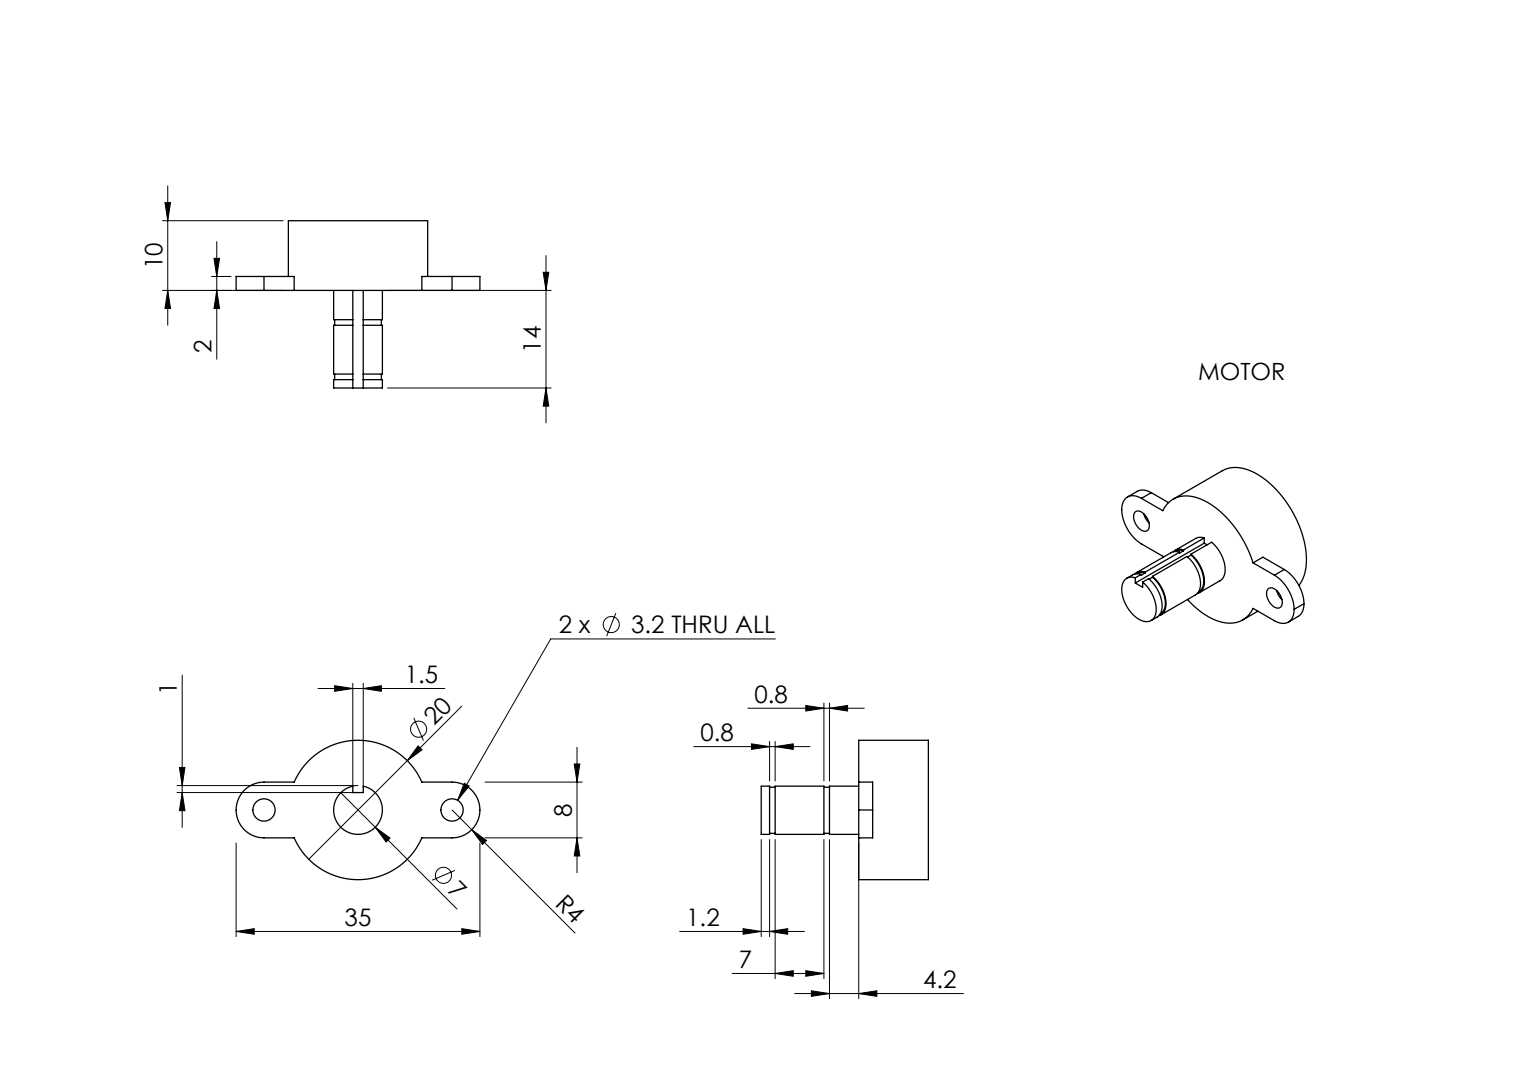
ISO-10303-21;
HEADER;
FILE_DESCRIPTION (('STEP AP214'),
    '1' );
FILE_NAME ('motor.step',
    '2026-10-26T05:17:54',
    ( '' ),
    ( '' ),
    'SwSTEP 2.0',
    'SolidWorks 2026',
    '' );
FILE_SCHEMA (( 'AUTOMOTIVE_DESIGN' ));
ENDSEC;

DATA;
#3=ORIENTED_EDGE ( 'NONE', *, *, #1888, .T. ) ;
#13=CARTESIAN_POINT ( 'NONE',  ( 19.89999999999999503, 90.00000000000000000, -8.000000000000000000 ) ) ;
#19=EDGE_CURVE ( 'NONE', #6404, #5937, #10592, .T. ) ;
#21=CIRCLE ( 'NONE', #6519, 3.500000000000003109 ) ;
#29=VERTEX_POINT ( 'NONE', #4640 ) ;
#47=ORIENTED_EDGE ( 'NONE', *, *, #5628, .T. ) ;
#48=EDGE_CURVE ( 'NONE', #8414, #6329, #6123, .T. ) ;
#56=PLANE ( 'NONE',  #9383 ) ;
#67=DIRECTION ( 'NONE',  ( 0.000000000000000000, 1.000000000000000000, 0.000000000000000000 ) ) ;
#70=LINE ( 'NONE', #8139, #12259 ) ;
#71=ORIENTED_EDGE ( 'NONE', *, *, #3443, .T. ) ;
#83=AXIS2_PLACEMENT_3D ( 'NONE', #3379, #1527, #7355 ) ;
#88=ORIENTED_EDGE ( 'NONE', *, *, #8982, .F. ) ;
#103=CIRCLE ( 'NONE', #2000, 3.500000000000003109 ) ;
#107=DIRECTION ( 'NONE',  ( -1.000000000000000000, 0.000000000000000000, 0.000000000000000000 ) ) ;
#115=VECTOR ( 'NONE', #5469, 1000.000000000000000 ) ;
#121=DIRECTION ( 'NONE',  ( -0.8665440819333538602, -0.4991005450470686888, -4.805464830191153728E-17 ) ) ;
#126=ORIENTED_EDGE ( 'NONE', *, *, #19, .T. ) ;
#142=DIRECTION ( 'NONE',  ( -0.000000000000000000, 0.000000000000000000, -1.000000000000000000 ) ) ;
#145=CARTESIAN_POINT ( 'NONE',  ( 34.25000000000000000, 92.49999999999998579, 4.800000000000000711 ) ) ;
#151=ORIENTED_EDGE ( 'NONE', *, *, #731, .F. ) ;
#165=AXIS2_PLACEMENT_3D ( 'NONE', #5058, #1689, #12557 ) ;
#166=LINE ( 'NONE', #6266, #6322 ) ;
#170=PRODUCT_DEFINITION_CONTEXT ( 'detailed design', #1838, 'design' ) ;
#181=ORIENTED_EDGE ( 'NONE', *, *, #7547, .F. ) ;
#185=DIRECTION ( 'NONE',  ( -0.3553942263724512163, 0.9347165045408831752, 0.000000000000000000 ) ) ;
#187=DIRECTION ( 'NONE',  ( -0.000000000000000000, -0.000000000000000000, -1.000000000000000000 ) ) ;
#191=VERTEX_POINT ( 'NONE', #1882 ) ;
#216=VERTEX_POINT ( 'NONE', #11026 ) ;
#237=VERTEX_POINT ( 'NONE', #12343 ) ;
#250=CARTESIAN_POINT ( 'NONE',  ( 50.09999999999995168, 90.00000000000000000, -10.00000000000000000 ) ) ;
#251=FACE_OUTER_BOUND ( 'NONE', #2972, .T. ) ;
#252=VERTEX_POINT ( 'NONE', #288 ) ;
#285=DIRECTION ( 'NONE',  ( 0.000000000000000000, 0.000000000000000000, -1.000000000000000000 ) ) ;
#288=CARTESIAN_POINT ( 'NONE',  ( 50.09999999999995168, 90.00000000000000000, -8.000000000000000000 ) ) ;
#292=CARTESIAN_POINT ( 'NONE',  ( 35.00000000000000000, 90.00000000000000000, 4.000000000000000000 ) ) ;
#294=VERTEX_POINT ( 'NONE', #6118 ) ;
#297=CARTESIAN_POINT ( 'NONE',  ( 52.49999999999996447, 94.00000000000000000, -10.00000000000000000 ) ) ;
#299=ORIENTED_EDGE ( 'NONE', *, *, #12486, .F. ) ;
#310=EDGE_CURVE ( 'NONE', #8511, #12562, #11290, .T. ) ;
#337=DIRECTION ( 'NONE',  ( -0.000000000000000000, -0.000000000000000000, -1.000000000000000000 ) ) ;
#341=DIRECTION ( 'NONE',  ( -0.3262398754384822630, 0.9452870165584014162, 0.000000000000000000 ) ) ;
#358=AXIS2_PLACEMENT_3D ( 'NONE', #3613, #12439, #9423 ) ;
#370=VERTEX_POINT ( 'NONE', #1148 ) ;
#387=ORIENTED_EDGE ( 'NONE', *, *, #9281, .T. ) ;
#393=CIRCLE ( 'NONE', #7723, 4.000000000000003553 ) ;
#400=AXIS2_PLACEMENT_3D ( 'NONE', #292, #2539, #8422 ) ;
#401=CARTESIAN_POINT ( 'NONE',  ( 48.49999999999995737, 94.00000000000000000, -8.000000000000000000 ) ) ;
#403=CARTESIAN_POINT ( 'NONE',  ( 35.00000000000000000, 90.00000000000000000, 4.800000000000000711 ) ) ;
#407=ADVANCED_FACE ( 'NONE', ( #2595 ), #7436, .F. ) ;
#408=VERTEX_POINT ( 'NONE', #12543 ) ;
#409=CARTESIAN_POINT ( 'NONE',  ( 25.00000000000000000, 90.00000000000000000, -10.00000000000000000 ) ) ;
#412=ORIENTED_EDGE ( 'NONE', *, *, #1216, .T. ) ;
#430=DIRECTION ( 'NONE',  ( -5.624500927088228034E-17, 1.370729058197317775E-18, 1.000000000000000000 ) ) ;
#431=AXIS2_PLACEMENT_3D ( 'NONE', #2573, #8714, #3560 ) ;
#447=DIRECTION ( 'NONE',  ( 0.000000000000000000, 0.000000000000000000, -1.000000000000000000 ) ) ;
#457=AXIS2_PLACEMENT_3D ( 'NONE', #11629, #9541, #8624 ) ;
#463=DIRECTION ( 'NONE',  ( -0.000000000000000000, -0.000000000000000000, 1.000000000000000000 ) ) ;
#485=VERTEX_POINT ( 'NONE', #3968 ) ;
#499=AXIS2_PLACEMENT_3D ( 'NONE', #6594, #5619, #11504 ) ;
#507=LINE ( 'NONE', #4515, #8154 ) ;
#531=EDGE_CURVE ( 'NONE', #3957, #12821, #1005, .T. ) ;
#535=DIRECTION ( 'NONE',  ( -5.624500927088228034E-17, 1.370729058197317968E-18, 1.000000000000000000 ) ) ;
#537=LINE ( 'NONE', #1464, #10952 ) ;
#543=ORIENTED_EDGE ( 'NONE', *, *, #11638, .F. ) ;
#557=ORIENTED_EDGE ( 'NONE', *, *, #7447, .F. ) ;
#565=FACE_OUTER_BOUND ( 'NONE', #1775, .T. ) ;
#575=ORIENTED_EDGE ( 'NONE', *, *, #4120, .F. ) ;
#578=ORIENTED_EDGE ( 'NONE', *, *, #7988, .T. ) ;
#581=AXIS2_PLACEMENT_3D ( 'NONE', #6283, #2043, #10989 ) ;
#583=DIRECTION ( 'NONE',  ( -1.000000000000000000, 0.000000000000000000, 0.000000000000000000 ) ) ;
#600=AXIS2_PLACEMENT_3D ( 'NONE', #4155, #337, #1325 ) ;
#624=AXIS2_PLACEMENT_3D ( 'NONE', #12004, #1206, #5133 ) ;
#636=CARTESIAN_POINT ( 'NONE',  ( 35.75000000000000711, 92.49999999999998579, -3.000000000000000000 ) ) ;
#644=ORIENTED_EDGE ( 'NONE', *, *, #5801, .F. ) ;
#650=ORIENTED_EDGE ( 'NONE', *, *, #2075, .F. ) ;
#655=VERTEX_POINT ( 'NONE', #9185 ) ;
#660=FACE_OUTER_BOUND ( 'NONE', #1254, .T. ) ;
#668=DIRECTION ( 'NONE',  ( 0.000000000000000000, 1.000000000000000000, -1.370729058197317775E-18 ) ) ;
#675=DIRECTION ( 'NONE',  ( 5.624500927088228034E-17, -1.370729058197317775E-18, -1.000000000000000000 ) ) ;
#681=VERTEX_POINT ( 'NONE', #7030 ) ;
#693=EDGE_CURVE ( 'NONE', #12083, #4963, #12636, .T. ) ;
#699=CLOSED_SHELL ( 'NONE', ( #4681, #2294, #5712, #12137, #6395, #6284, #10454, #6271, #7033, #8769, #9664, #6996, #3078, #6506, #5758, #9872, #10478, #5588, #2469, #1397, #4829, #5175, #6473, #11028, #2843, #8926, #11939, #3918, #407, #9755, #9220, #11801, #9117, #7996, #2544, #5940, #1715, #12395, #866, #5366, #1669, #7054, #12542, #2318, #6182, #10197, #10507 ) ) ;
#705=EDGE_CURVE ( 'NONE', #12083, #370, #10296, .T. ) ;
#706=ORIENTED_EDGE ( 'NONE', *, *, #3432, .T. ) ;
#719=FACE_OUTER_BOUND ( 'NONE', #6790, .T. ) ;
#721=CIRCLE ( 'NONE', #499, 10.00000000000000178 ) ;
#731=EDGE_CURVE ( 'NONE', #10645, #11257, #10099, .T. ) ;
#738=CARTESIAN_POINT ( 'NONE',  ( 31.50000000000000000, 90.00000000000000000, -8.000000000000000000 ) ) ;
#769=CARTESIAN_POINT ( 'NONE',  ( 34.25000000000000000, 92.49999999999998579, 4.000000000000000000 ) ) ;
#777=DIRECTION ( 'NONE',  ( 0.4719909656437444867, -0.8816033849473842166, 0.000000000000000000 ) ) ;
#781=ORIENTED_EDGE ( 'NONE', *, *, #10591, .T. ) ;
#785=CIRCLE ( 'NONE', #2474, 3.500000000000003109 ) ;
#796=DIRECTION ( 'NONE',  ( -0.3262398754384820410, 0.9452870165584015272, 0.000000000000000000 ) ) ;
#806=ORIENTED_EDGE ( 'NONE', *, *, #5628, .F. ) ;
#811=LINE ( 'NONE', #3838, #1160 ) ;
#823=DIRECTION ( 'NONE',  ( -0.000000000000000000, 0.000000000000000000, 1.000000000000000000 ) ) ;
#839=AXIS2_PLACEMENT_3D ( 'NONE', #8214, #8409, #1467 ) ;
#840=CARTESIAN_POINT ( 'NONE',  ( 19.89999999999999503, 90.00000000000000000, -10.00000000000000000 ) ) ;
#841=EDGE_CURVE ( 'NONE', #3363, #7515, #10366, .T. ) ;
#843=LINE ( 'NONE', #2699, #6376 ) ;
#849=ORIENTED_EDGE ( 'NONE', *, *, #1595, .F. ) ;
#866=ADVANCED_FACE ( 'NONE', ( #2390 ), #7550, .T. ) ;
#867=EDGE_CURVE ( 'NONE', #12412, #10917, #6497, .T. ) ;
#869=LINE ( 'NONE', #9776, #11647 ) ;
#879=AXIS2_PLACEMENT_3D ( 'NONE', #12949, #12888, #6862 ) ;
#885=CARTESIAN_POINT ( 'NONE',  ( 21.49999999999998579, 90.00000000000000000, -10.00000000000000000 ) ) ;
#888=ORIENTED_EDGE ( 'NONE', *, *, #8720, .T. ) ;
#898=( GEOMETRIC_REPRESENTATION_CONTEXT ( 3 ) GLOBAL_UNCERTAINTY_ASSIGNED_CONTEXT ( ( #6165 ) ) GLOBAL_UNIT_ASSIGNED_CONTEXT ( ( #7994, #6701, #11056 ) ) REPRESENTATION_CONTEXT ( 'NONE', 'WORKASPACE' ) );
#914=VECTOR ( 'NONE', #1674, 1000.000000000000000 ) ;
#917=EDGE_CURVE ( 'NONE', #12608, #8631, #537, .T. ) ;
#931=EDGE_CURVE ( 'NONE', #1668, #8414, #9445, .T. ) ;
#934=AXIS2_PLACEMENT_3D ( 'NONE', #10445, #11553, #3520 ) ;
#938=EDGE_CURVE ( 'NONE', #252, #6072, #5110, .T. ) ;
#971=DIRECTION ( 'NONE',  ( -0.000000000000000000, -0.000000000000000000, -1.000000000000000000 ) ) ;
#980=CIRCLE ( 'NONE', #9970, 4.000000000000000000 ) ;
#981=DIRECTION ( 'NONE',  ( -0.000000000000000000, -0.000000000000000000, 1.000000000000000000 ) ) ;
#993=DIRECTION ( 'NONE',  ( 1.000000000000000000, 0.000000000000000000, 0.000000000000000000 ) ) ;
#1005=LINE ( 'NONE', #10886, #10745 ) ;
#1012=AXIS2_PLACEMENT_3D ( 'NONE', #9319, #2389, #5259 ) ;
#1020=DIRECTION ( 'NONE',  ( 0.000000000000000000, 0.000000000000000000, 1.000000000000000000 ) ) ;
#1026=ORIENTED_EDGE ( 'NONE', *, *, #5667, .T. ) ;
#1042=VECTOR ( 'NONE', #2332, 1000.000000000000000 ) ;
#1043=CARTESIAN_POINT ( 'NONE',  ( 17.49999999999998579, 90.00000000000002842, -8.000000000000000000 ) ) ;
#1072=DIRECTION ( 'NONE',  ( -1.000000000000000000, 0.000000000000000000, 0.000000000000000000 ) ) ;
#1074=ORIENTED_EDGE ( 'NONE', *, *, #9115, .T. ) ;
#1087=CIRCLE ( 'NONE', #457, 1.599999999999990319 ) ;
#1099=ORIENTED_EDGE ( 'NONE', *, *, #12396, .F. ) ;
#1124=DIRECTION ( 'NONE',  ( 0.000000000000000000, 1.000000000000000000, -1.370729058197317775E-18 ) ) ;
#1126=ORIENTED_EDGE ( 'NONE', *, *, #8124, .T. ) ;
#1128=FACE_OUTER_BOUND ( 'NONE', #1276, .T. ) ;
#1136=LINE ( 'NONE', #145, #7950 ) ;
#1141=AXIS2_PLACEMENT_3D ( 'NONE', #1428, #3600, #12425 ) ;
#1148=CARTESIAN_POINT ( 'NONE',  ( 33.90709641728108892, 93.16671150547063007, 4.000000000000000000 ) ) ;
#1158=EDGE_LOOP ( 'NONE', ( #7100, #8756, #5861, #11911, #2951, #5490, #7151, #3080, #5486, #5090, #126, #8702 ) ) ;
#1160=VECTOR ( 'NONE', #10888, 1000.000000000000000 ) ;
#1166=EDGE_LOOP ( 'NONE', ( #412, #7388 ) ) ;
#1169=PRODUCT_CONTEXT ( 'NONE', #10180, 'mechanical' ) ;
#1180=LINE ( 'NONE', #250, #9978 ) ;
#1183=CARTESIAN_POINT ( 'NONE',  ( 35.00000000000000000, 90.00000000000000000, 6.000000000000000000 ) ) ;
#1206=DIRECTION ( 'NONE',  ( -0.000000000000000000, -0.000000000000000000, -1.000000000000000000 ) ) ;
#1211=CARTESIAN_POINT ( 'NONE',  ( 34.25000000000000000, 93.41869858279433458, 4.800000000000000711 ) ) ;
#1216=EDGE_CURVE ( 'NONE', #1668, #4783, #721, .T. ) ;
#1220=CARTESIAN_POINT ( 'NONE',  ( 35.00000000000000000, 90.00000000000000000, 4.000000000000000000 ) ) ;
#1222=ORIENTED_EDGE ( 'NONE', *, *, #48, .F. ) ;
#1223=DIRECTION ( 'NONE',  ( 5.624500927088228034E-17, -1.370729058197317775E-18, -1.000000000000000000 ) ) ;
#1231=ORIENTED_EDGE ( 'NONE', *, *, #5801, .T. ) ;
#1235=CIRCLE ( 'NONE', #10439, 3.349999999999995204 ) ;
#1236=DIRECTION ( 'NONE',  ( 0.000000000000000000, 0.000000000000000000, 1.000000000000000000 ) ) ;
#1254=EDGE_LOOP ( 'NONE', ( #7238, #10734, #387, #7725 ) ) ;
#1257=AXIS2_PLACEMENT_3D ( 'NONE', #12940, #5020, #6193 ) ;
#1274=DIRECTION ( 'NONE',  ( -0.9549484348006339607, -0.2967717757331703732, 0.000000000000000000 ) ) ;
#1276=EDGE_LOOP ( 'NONE', ( #4208, #71, #3279, #2759 ) ) ;
#1289=LINE ( 'NONE', #6262, #7232 ) ;
#1296=ORIENTED_EDGE ( 'NONE', *, *, #3497, .F. ) ;
#1299=CARTESIAN_POINT ( 'NONE',  ( 52.49999999999996447, 90.00000000000000000, -10.00000000000000000 ) ) ;
#1311=DIRECTION ( 'NONE',  ( 5.624500927088228034E-17, -1.370729058197317775E-18, -1.000000000000000000 ) ) ;
#1325=DIRECTION ( 'NONE',  ( -1.000000000000000000, 0.000000000000000000, 0.000000000000000000 ) ) ;
#1335=ORIENTED_EDGE ( 'NONE', *, *, #5063, .F. ) ;
#1343=LINE ( 'NONE', #9197, #12715 ) ;
#1348=FACE_OUTER_BOUND ( 'NONE', #2904, .T. ) ;
#1353=VERTEX_POINT ( 'NONE', #7583 ) ;
#1357=CIRCLE ( 'NONE', #12227, 3.500000000000003109 ) ;
#1363=ORIENTED_EDGE ( 'NONE', *, *, #917, .F. ) ;
#1371=DIRECTION ( 'NONE',  ( 0.000000000000000000, -0.000000000000000000, 1.000000000000000000 ) ) ;
#1372=ORIENTED_EDGE ( 'NONE', *, *, #6536, .T. ) ;
#1381=ORIENTED_EDGE ( 'NONE', *, *, #6577, .T. ) ;
#1392=DIRECTION ( 'NONE',  ( -0.000000000000000000, -0.000000000000000000, -1.000000000000000000 ) ) ;
#1397=ADVANCED_FACE ( 'NONE', ( #2997 ), #11830, .F. ) ;
#1405=DIRECTION ( 'NONE',  ( -1.000000000000000000, 0.000000000000000000, 0.000000000000000000 ) ) ;
#1414=DIRECTION ( 'NONE',  ( -1.000000000000000000, 0.000000000000000000, 0.000000000000000000 ) ) ;
#1428=CARTESIAN_POINT ( 'NONE',  ( 35.00000000000000000, 90.00000000000000000, 4.800000000000000711 ) ) ;
#1443=AXIS2_PLACEMENT_3D ( 'NONE', #5383, #142, #7228 ) ;
#1448=ORIENTED_EDGE ( 'NONE', *, *, #3532, .F. ) ;
#1464=CARTESIAN_POINT ( 'NONE',  ( 34.25000000000000000, 92.49999999999998579, -3.799999999999999378 ) ) ;
#1467=DIRECTION ( 'NONE',  ( 1.000000000000000000, 0.000000000000000000, 0.000000000000000000 ) ) ;
#1469=ORIENTED_EDGE ( 'NONE', *, *, #11376, .T. ) ;
#1487=DIRECTION ( 'NONE',  ( -0.3262398754384822630, 0.9452870165584014162, 0.000000000000000000 ) ) ;
#1489=EDGE_CURVE ( 'NONE', #191, #4989, #6156, .T. ) ;
#1503=EDGE_CURVE ( 'NONE', #6072, #252, #4507, .T. ) ;
#1527=DIRECTION ( 'NONE',  ( 0.000000000000000000, 0.000000000000000000, -1.000000000000000000 ) ) ;
#1530=CARTESIAN_POINT ( 'NONE',  ( 25.83484861008832567, 94.00000000000000000, -18.00000000000000355 ) ) ;
#1552=DIRECTION ( 'NONE',  ( 0.000000000000000000, -0.000000000000000000, 1.000000000000000000 ) ) ;
#1554=DIRECTION ( 'NONE',  ( -0.000000000000000000, -0.000000000000000000, 1.000000000000000000 ) ) ;
#1567=ORIENTED_EDGE ( 'NONE', *, *, #1605, .F. ) ;
#1570=LINE ( 'NONE', #2625, #7138 ) ;
#1572=ORIENTED_EDGE ( 'NONE', *, *, #5667, .F. ) ;
#1577=ORIENTED_EDGE ( 'NONE', *, *, #9238, .F. ) ;
#1595=EDGE_CURVE ( 'NONE', #191, #7314, #8165, .T. ) ;
#1605=EDGE_CURVE ( 'NONE', #2737, #4447, #9508, .T. ) ;
#1612=CARTESIAN_POINT ( 'NONE',  ( 34.25000000000000000, 92.49999999999998579, -9.802775637731997449 ) ) ;
#1624=CARTESIAN_POINT ( 'NONE',  ( 32.09707732552327286, 88.32801317409231956, -3.800000000000000266 ) ) ;
#1625=EDGE_CURVE ( 'NONE', #8631, #6452, #1357, .T. ) ;
#1630=ORIENTED_EDGE ( 'NONE', *, *, #1964, .F. ) ;
#1637=EDGE_CURVE ( 'NONE', #12207, #7597, #3676, .T. ) ;
#1641=DIRECTION ( 'NONE',  ( -0.000000000000000000, -0.000000000000000000, -1.000000000000000000 ) ) ;
#1656=VECTOR ( 'NONE', #1725, 1000.000000000000000 ) ;
#1658=AXIS2_PLACEMENT_3D ( 'NONE', #12179, #4204, #2310 ) ;
#1661=LINE ( 'NONE', #6561, #5018 ) ;
#1668=VERTEX_POINT ( 'NONE', #7174 ) ;
#1669=ADVANCED_FACE ( 'NONE', ( #1348 ), #2217, .F. ) ;
#1674=DIRECTION ( 'NONE',  ( 0.000000000000000000, -1.000000000000000000, 1.370729058197317775E-18 ) ) ;
#1689=DIRECTION ( 'NONE',  ( -5.624500927088228034E-17, 1.370729058197317968E-18, 1.000000000000000000 ) ) ;
#1694=VERTEX_POINT ( 'NONE', #4753 ) ;
#1706=DIRECTION ( 'NONE',  ( 0.000000000000000000, 0.000000000000000000, -1.000000000000000000 ) ) ;
#1712=CARTESIAN_POINT ( 'NONE',  ( 34.25000000000000000, 93.41869858279433458, 4.000000000000000000 ) ) ;
#1715=ADVANCED_FACE ( 'NONE', ( #5601 ), #9718, .F. ) ;
#1724=EDGE_CURVE ( 'NONE', #6762, #12412, #3252, .T. ) ;
#1725=DIRECTION ( 'NONE',  ( -0.000000000000000000, -0.000000000000000000, -1.000000000000000000 ) ) ;
#1735=VERTEX_POINT ( 'NONE', #3711 ) ;
#1746=EDGE_LOOP ( 'NONE', ( #9745, #2949, #5116, #2908, #10024, #12272 ) ) ;
#1754=ORIENTED_EDGE ( 'NONE', *, *, #5511, .F. ) ;
#1767=CARTESIAN_POINT ( 'NONE',  ( 35.00000000000000000, 90.00000000000000000, -3.000000000000000000 ) ) ;
#1769=AXIS2_PLACEMENT_3D ( 'NONE', #403, #2652, #8472 ) ;
#1774=DIRECTION ( 'NONE',  ( -0.3262398754384820410, 0.9452870165584015272, 0.000000000000000000 ) ) ;
#1775=EDGE_LOOP ( 'NONE', ( #3619, #4581, #9169, #3707 ) ) ;
#1777=DIRECTION ( 'NONE',  ( -0.000000000000000000, -0.000000000000000000, -1.000000000000000000 ) ) ;
#1789=VECTOR ( 'NONE', #4577, 1000.000000000000000 ) ;
#1797=ORIENTED_EDGE ( 'NONE', *, *, #731, .T. ) ;
#1816=DIRECTION ( 'NONE',  ( -5.624500927088228034E-17, 1.370729058197317775E-18, 1.000000000000000000 ) ) ;
#1817=CARTESIAN_POINT ( 'NONE',  ( 35.00000000000000000, 90.00000000000000000, 4.000000000000000000 ) ) ;
#1828=ORIENTED_EDGE ( 'NONE', *, *, #4046, .T. ) ;
#1830=VERTEX_POINT ( 'NONE', #5004 ) ;
#1838=APPLICATION_CONTEXT ( 'automotive_design' ) ;
#1870=CIRCLE ( 'NONE', #9177, 3.350000000000003642 ) ;
#1875=EDGE_CURVE ( 'NONE', #10645, #1694, #6587, .T. ) ;
#1877=VECTOR ( 'NONE', #11062, 1000.000000000000000 ) ;
#1882=CARTESIAN_POINT ( 'NONE',  ( 38.50000000000000711, 90.00000000000000000, 4.000000000000000000 ) ) ;
#1883=CIRCLE ( 'NONE', #2727, 4.000000000000000000 ) ;
#1888=EDGE_CURVE ( 'NONE', #408, #2123, #103, .T. ) ;
#1914=ORIENTED_EDGE ( 'NONE', *, *, #8639, .T. ) ;
#1920=FACE_OUTER_BOUND ( 'NONE', #12041, .T. ) ;
#1936=ORIENTED_EDGE ( 'NONE', *, *, #8160, .F. ) ;
#1950=ORIENTED_EDGE ( 'NONE', *, *, #9238, .T. ) ;
#1955=ORIENTED_EDGE ( 'NONE', *, *, #1605, .T. ) ;
#1956=CARTESIAN_POINT ( 'NONE',  ( 34.25000000000000000, 93.41869858279433458, -3.000000000000000888 ) ) ;
#1959=STYLED_ITEM ( 'NONE', ( #8256 ), #8095 ) ;
#1964=EDGE_CURVE ( 'NONE', #2737, #10645, #811, .T. ) ;
#1968=DIRECTION ( 'NONE',  ( 0.000000000000000000, 0.000000000000000000, -1.000000000000000000 ) ) ;
#1981=ORIENTED_EDGE ( 'NONE', *, *, #4046, .F. ) ;
#1984=CARTESIAN_POINT ( 'NONE',  ( 34.25000000000000000, 93.26496554346289258, 4.800000000000000711 ) ) ;
#1988=DIRECTION ( 'NONE',  ( -5.624500927088228034E-17, 1.370729058197317775E-18, 1.000000000000000000 ) ) ;
#2000=AXIS2_PLACEMENT_3D ( 'NONE', #9846, #3907, #7032 ) ;
#2005=CARTESIAN_POINT ( 'NONE',  ( 31.50000000000000000, 90.00000000000000000, 6.000000000000000000 ) ) ;
#2010=DIRECTION ( 'NONE',  ( -0.000000000000000000, -0.000000000000000000, -1.000000000000000000 ) ) ;
#2023=DIRECTION ( 'NONE',  ( -0.3262398754384822630, 0.9452870165584014162, 0.000000000000000000 ) ) ;
#2026=DIRECTION ( 'NONE',  ( 5.624500927088228034E-17, -1.370729058197317775E-18, -1.000000000000000000 ) ) ;
#2037=EDGE_LOOP ( 'NONE', ( #575, #9948, #11098, #3, #1099, #1754 ) ) ;
#2043=DIRECTION ( 'NONE',  ( 0.000000000000000000, 0.000000000000000000, -1.000000000000000000 ) ) ;
#2055=LINE ( 'NONE', #7149, #8796 ) ;
#2064=DIRECTION ( 'NONE',  ( 0.000000000000000000, -0.000000000000000000, 1.000000000000000000 ) ) ;
#2068=DIRECTION ( 'NONE',  ( -1.000000000000000000, 0.000000000000000000, -0.000000000000000000 ) ) ;
#2074=CIRCLE ( 'NONE', #1443, 4.000000000000000000 ) ;
#2075=EDGE_CURVE ( 'NONE', #3524, #1694, #2330, .T. ) ;
#2091=DIRECTION ( 'NONE',  ( 0.4719909656437444867, -0.8816033849473842166, 0.000000000000000000 ) ) ;
#2103=ORIENTED_EDGE ( 'NONE', *, *, #10688, .T. ) ;
#2108=CARTESIAN_POINT ( 'NONE',  ( 35.00000000000000000, 90.00000000000000000, 4.800000000000000711 ) ) ;
#2110=DIRECTION ( 'NONE',  ( -0.8665440819333538602, -0.4991005450470686888, -4.805464830191153728E-17 ) ) ;
#2123=VERTEX_POINT ( 'NONE', #4227 ) ;
#2131=AXIS2_PLACEMENT_3D ( 'NONE', #7843, #10790, #2023 ) ;
#2133=FACE_OUTER_BOUND ( 'NONE', #10319, .T. ) ;
#2137=ORIENTED_EDGE ( 'NONE', *, *, #5023, .F. ) ;
#2145=CARTESIAN_POINT ( 'NONE',  ( 35.00000000000000000, 90.00000000000000000, -3.799999999999999378 ) ) ;
#2147=ORIENTED_EDGE ( 'NONE', *, *, #12555, .F. ) ;
#2148=AXIS2_PLACEMENT_3D ( 'NONE', #11822, #5987, #2990 ) ;
#2152=EDGE_LOOP ( 'NONE', ( #6828, #7770, #5880, #2183, #806, #9980 ) ) ;
#2176=CARTESIAN_POINT ( 'NONE',  ( 21.49999999999998579, 86.00000000000000000, -10.00000000000000000 ) ) ;
#2177=VERTEX_POINT ( 'NONE', #3572 ) ;
#2183=ORIENTED_EDGE ( 'NONE', *, *, #9832, .F. ) ;
#2185=DIRECTION ( 'NONE',  ( 0.4719909656437442647, -0.8816033849473842166, 2.775557561595757269E-17 ) ) ;
#2207=CARTESIAN_POINT ( 'NONE',  ( 48.49999999999995737, 90.00000000000000000, -10.00000000000000000 ) ) ;
#2217=PLANE ( 'NONE',  #4496 ) ;
#2225=CIRCLE ( 'NONE', #4933, 3.500000000000003109 ) ;
#2231=ORIENTED_EDGE ( 'NONE', *, *, #6103, .T. ) ;
#2237=ORIENTED_EDGE ( 'NONE', *, *, #12195, .F. ) ;
#2244=DIRECTION ( 'NONE',  ( 0.000000000000000000, 1.000000000000000000, 0.000000000000000000 ) ) ;
#2253=EDGE_LOOP ( 'NONE', ( #9736, #12024, #1577, #9723 ) ) ;
#2265=CARTESIAN_POINT ( 'NONE',  ( 52.49999999999996447, 94.00000000000000000, -10.00000000000000000 ) ) ;
#2269=EDGE_CURVE ( 'NONE', #12412, #8709, #8408, .T. ) ;
#2273=VECTOR ( 'NONE', #9361, 1000.000000000000000 ) ;
#2289=ORIENTED_EDGE ( 'NONE', *, *, #1637, .T. ) ;
#2293=ORIENTED_EDGE ( 'NONE', *, *, #11013, .F. ) ;
#2294=ADVANCED_FACE ( 'NONE', ( #9642 ), #7422, .F. ) ;
#2310=DIRECTION ( 'NONE',  ( 1.000000000000000000, 0.000000000000000000, -0.000000000000000000 ) ) ;
#2318=ADVANCED_FACE ( 'NONE', ( #8473 ), #12461, .T. ) ;
#2330=LINE ( 'NONE', #6108, #7434 ) ;
#2332=DIRECTION ( 'NONE',  ( 1.000000000000000000, -0.000000000000000000, -0.000000000000000000 ) ) ;
#2335=EDGE_CURVE ( 'NONE', #4130, #7314, #2225, .T. ) ;
#2339=CARTESIAN_POINT ( 'NONE',  ( 23.09999999999997300, 90.00000000000000000, -10.00000000000000000 ) ) ;
#2344=FACE_OUTER_BOUND ( 'NONE', #10064, .T. ) ;
#2346=CARTESIAN_POINT ( 'NONE',  ( 35.00000000000000000, 90.00000000000000000, -3.799999999999999822 ) ) ;
#2349=PRODUCT_DEFINITION ( 'UNKNOWN', '', #6557, #170 ) ;
#2352=DIRECTION ( 'NONE',  ( -5.624500927088228034E-17, 1.370729058197317775E-18, 1.000000000000000000 ) ) ;
#2361=ORIENTED_EDGE ( 'NONE', *, *, #10556, .T. ) ;
#2378=VERTEX_POINT ( 'NONE', #738 ) ;
#2389=DIRECTION ( 'NONE',  ( 0.000000000000000000, 0.000000000000000000, -1.000000000000000000 ) ) ;
#2390=FACE_OUTER_BOUND ( 'NONE', #12019, .T. ) ;
#2406=EDGE_CURVE ( 'NONE', #11844, #11880, #12868, .T. ) ;
#2407=ORIENTED_EDGE ( 'NONE', *, *, #1637, .F. ) ;
#2409=DIRECTION ( 'NONE',  ( 0.000000000000000000, 0.000000000000000000, -1.000000000000000000 ) ) ;
#2410=DIRECTION ( 'NONE',  ( -0.000000000000000000, -0.000000000000000000, -1.000000000000000000 ) ) ;
#2415=ORIENTED_EDGE ( 'NONE', *, *, #9712, .F. ) ;
#2419=VERTEX_POINT ( 'NONE', #4990 ) ;
#2428=ORIENTED_EDGE ( 'NONE', *, *, #841, .F. ) ;
#2448=CARTESIAN_POINT ( 'NONE',  ( 34.25000000000000000, 92.49999999999998579, 6.000000000000000000 ) ) ;
#2449=VECTOR ( 'NONE', #8607, 1000.000000000000114 ) ;
#2454=DIRECTION ( 'NONE',  ( -0.3262398754384822630, 0.9452870165584014162, 0.000000000000000000 ) ) ;
#2457=DIRECTION ( 'NONE',  ( 0.000000000000000000, 1.000000000000000000, 0.000000000000000000 ) ) ;
#2460=LINE ( 'NONE', #4229, #4608 ) ;
#2464=LINE ( 'NONE', #2660, #12900 ) ;
#2469=ADVANCED_FACE ( 'NONE', ( #1920 ), #5901, .F. ) ;
#2474=AXIS2_PLACEMENT_3D ( 'NONE', #7848, #1706, #7658 ) ;
#2487=DIRECTION ( 'NONE',  ( 0.000000000000000000, 0.000000000000000000, 1.000000000000000000 ) ) ;
#2500=FACE_OUTER_BOUND ( 'NONE', #5926, .T. ) ;
#2539=DIRECTION ( 'NONE',  ( 0.000000000000000000, 0.000000000000000000, -1.000000000000000000 ) ) ;
#2544=ADVANCED_FACE ( 'NONE', ( #8266 ), #7216, .T. ) ;
#2546=CIRCLE ( 'NONE', #431, 3.500000000000003109 ) ;
#2548=EDGE_LOOP ( 'NONE', ( #8498, #47, #12554, #10610 ) ) ;
#2573=CARTESIAN_POINT ( 'NONE',  ( 35.00000000000000000, 90.00000000000000000, -3.799999999999999378 ) ) ;
#2577=CYLINDRICAL_SURFACE ( 'NONE', #10215, 10.00000000000000178 ) ;
#2580=CARTESIAN_POINT ( 'NONE',  ( 34.25000000000000000, 93.41869858279433458, 6.000000000000000000 ) ) ;
#2581=LINE ( 'NONE', #6431, #1656 ) ;
#2586=DIRECTION ( 'NONE',  ( 1.000000000000000000, 0.000000000000000000, 0.000000000000000000 ) ) ;
#2589=COLOUR_RGB ( '',0.8941176470588234615, 0.8941176470588234615, 0.8941176470588234615 ) ;
#2595=FACE_OUTER_BOUND ( 'NONE', #6007, .T. ) ;
#2604=DIRECTION ( 'NONE',  ( -0.000000000000000000, -0.000000000000000000, -1.000000000000000000 ) ) ;
#2622=ORIENTED_EDGE ( 'NONE', *, *, #3607, .F. ) ;
#2624=ORIENTED_EDGE ( 'NONE', *, *, #8393, .T. ) ;
#2625=CARTESIAN_POINT ( 'NONE',  ( 35.75000000000000711, 92.49999999999998579, -8.000000000000000000 ) ) ;
#2652=DIRECTION ( 'NONE',  ( 0.000000000000000000, 0.000000000000000000, -1.000000000000000000 ) ) ;
#2653=EDGE_CURVE ( 'NONE', #11634, #5783, #6740, .T. ) ;
#2660=CARTESIAN_POINT ( 'NONE',  ( 31.50000000000000000, 90.00000000000000000, 6.000000000000000000 ) ) ;
#2663=CARTESIAN_POINT ( 'NONE',  ( 19.89999999999999858, 90.00000000000000000, -10.00000000000000178 ) ) ;
#2666=VERTEX_POINT ( 'NONE', #11048 ) ;
#2674=ORIENTED_EDGE ( 'NONE', *, *, #8986, .T. ) ;
#2680=CIRCLE ( 'NONE', #11656, 3.500000000000003109 ) ;
#2699=CARTESIAN_POINT ( 'NONE',  ( 52.49999999999996447, 86.00000000000000000, -8.000000000000000000 ) ) ;
#2727=AXIS2_PLACEMENT_3D ( 'NONE', #10655, #10784, #9801 ) ;
#2737=VERTEX_POINT ( 'NONE', #11113 ) ;
#2739=ORIENTED_EDGE ( 'NONE', *, *, #10530, .T. ) ;
#2758=LINE ( 'NONE', #10724, #11241 ) ;
#2759=ORIENTED_EDGE ( 'NONE', *, *, #10639, .T. ) ;
#2777=DIRECTION ( 'NONE',  ( 0.000000000000000000, -0.000000000000000000, 1.000000000000000000 ) ) ;
#2779=CIRCLE ( 'NONE', #8003, 3.350000000000003642 ) ;
#2787=ORIENTED_EDGE ( 'NONE', *, *, #1489, .T. ) ;
#2792=DIRECTION ( 'NONE',  ( 0.000000000000000000, 0.000000000000000000, -1.000000000000000000 ) ) ;
#2796=CARTESIAN_POINT ( 'NONE',  ( 48.49999999999995737, 94.00000000000000000, -10.00000000000000000 ) ) ;
#2808=CARTESIAN_POINT ( 'NONE',  ( 35.00000000000000000, 90.00000000000000000, 6.000000000000000000 ) ) ;
#2843=ADVANCED_FACE ( 'NONE', ( #9796 ), #2992, .T. ) ;
#2847=EDGE_LOOP ( 'NONE', ( #1296, #12159, #9133, #10090 ) ) ;
#2855=EDGE_LOOP ( 'NONE', ( #10880, #2293, #2137, #9670 ) ) ;
#2865=ORIENTED_EDGE ( 'NONE', *, *, #1503, .T. ) ;
#2883=CYLINDRICAL_SURFACE ( 'NONE', #2131, 3.349999999999995204 ) ;
#2885=FACE_OUTER_BOUND ( 'NONE', #8367, .T. ) ;
#2887=CIRCLE ( 'NONE', #7257, 10.00000000000000178 ) ;
#2900=CARTESIAN_POINT ( 'NONE',  ( 23.09999999999997300, 90.00000000000000000, -10.00000000000000178 ) ) ;
#2904=EDGE_LOOP ( 'NONE', ( #7306, #10371, #9401, #8329, #6249 ) ) ;
#2908=ORIENTED_EDGE ( 'NONE', *, *, #8160, .T. ) ;
#2910=ORIENTED_EDGE ( 'NONE', *, *, #693, .T. ) ;
#2911=DIRECTION ( 'NONE',  ( 0.000000000000000000, 0.000000000000000000, 1.000000000000000000 ) ) ;
#2940=VERTEX_POINT ( 'NONE', #11887 ) ;
#2949=ORIENTED_EDGE ( 'NONE', *, *, #10700, .T. ) ;
#2951=ORIENTED_EDGE ( 'NONE', *, *, #12396, .T. ) ;
#2968=LINE ( 'NONE', #1984, #11678 ) ;
#2971=CARTESIAN_POINT ( 'NONE',  ( 35.00000000000000000, 90.00000000000000000, -3.000000000000000888 ) ) ;
#2972=EDGE_LOOP ( 'NONE', ( #6291, #3797, #12728, #2237, #1074, #5573, #781, #10453, #11927, #9042, #4114, #888, #12061, #3449, #5344, #4146, #849, #2787, #1828, #11545 ) ) ;
#2986=AXIS2_PLACEMENT_3D ( 'NONE', #11038, #2026, #2091 ) ;
#2990=DIRECTION ( 'NONE',  ( 1.000000000000000000, 0.000000000000000000, 0.000000000000000000 ) ) ;
#2992=CYLINDRICAL_SURFACE ( 'NONE', #10087, 4.000000000000000000 ) ;
#2997=FACE_OUTER_BOUND ( 'NONE', #12705, .T. ) ;
#3008=ORIENTED_EDGE ( 'NONE', *, *, #5699, .T. ) ;
#3019=VECTOR ( 'NONE', #4351, 1000.000000000000000 ) ;
#3033=AXIS2_PLACEMENT_3D ( 'NONE', #7800, #3952, #9766 ) ;
#3053=DIRECTION ( 'NONE',  ( 0.000000000000000000, 0.000000000000000000, 1.000000000000000000 ) ) ;
#3060=CIRCLE ( 'NONE', #5972, 3.350000000000003642 ) ;
#3077=CARTESIAN_POINT ( 'NONE',  ( 38.50000000000000711, 90.00000000000000000, -8.000000000000000000 ) ) ;
#3078=ADVANCED_FACE ( 'NONE', ( #3127 ), #6749, .T. ) ;
#3080=ORIENTED_EDGE ( 'NONE', *, *, #2269, .T. ) ;
#3094=CARTESIAN_POINT ( 'NONE',  ( 31.86464806177570352, 88.44450386581220869, -3.000000000000000888 ) ) ;
#3096=CARTESIAN_POINT ( 'NONE',  ( 32.09707732552327286, 88.32801317409231956, -3.800000000000000266 ) ) ;
#3099=CARTESIAN_POINT ( 'NONE',  ( 17.49999999999998579, 90.00000000000002842, -10.00000000000000000 ) ) ;
#3127=FACE_OUTER_BOUND ( 'NONE', #4038, .T. ) ;
#3147=ORIENTED_EDGE ( 'NONE', *, *, #12775, .F. ) ;
#3179=DIRECTION ( 'NONE',  ( 0.000000000000000000, 0.000000000000000000, 1.000000000000000000 ) ) ;
#3180=EDGE_CURVE ( 'NONE', #11942, #3524, #11188, .T. ) ;
#3181=DIRECTION ( 'NONE',  ( 0.000000000000000000, 0.000000000000000000, 1.000000000000000000 ) ) ;
#3191=AXIS2_PLACEMENT_3D ( 'NONE', #3627, #8780, #12773 ) ;
#3195=DIRECTION ( 'NONE',  ( -5.624500927088228034E-17, 1.370729058197317775E-18, 1.000000000000000000 ) ) ;
#3226=SURFACE_STYLE_FILL_AREA ( #11739 ) ;
#3228=EDGE_CURVE ( 'NONE', #9676, #1830, #6509, .T. ) ;
#3231=ORIENTED_EDGE ( 'NONE', *, *, #9024, .F. ) ;
#3248=CARTESIAN_POINT ( 'NONE',  ( 48.49999999999995737, 90.00000000000000000, -10.00000000000000000 ) ) ;
#3252=CIRCLE ( 'NONE', #934, 3.349999999999995204 ) ;
#3254=ORIENTED_EDGE ( 'NONE', *, *, #1724, .T. ) ;
#3272=DIRECTION ( 'NONE',  ( 0.000000000000000000, -0.000000000000000000, 1.000000000000000000 ) ) ;
#3274=ORIENTED_EDGE ( 'NONE', *, *, #4879, .F. ) ;
#3278=LINE ( 'NONE', #8501, #8740 ) ;
#3279=ORIENTED_EDGE ( 'NONE', *, *, #10746, .T. ) ;
#3297=ORIENTED_EDGE ( 'NONE', *, *, #5990, .T. ) ;
#3305=CARTESIAN_POINT ( 'NONE',  ( 44.16515138991168499, 86.00000000000000000, -10.00000000000000000 ) ) ;
#3352=CARTESIAN_POINT ( 'NONE',  ( 35.75000000000000711, 92.49999999999998579, -9.802775637731997449 ) ) ;
#3363=VERTEX_POINT ( 'NONE', #9006 ) ;
#3364=AXIS2_PLACEMENT_3D ( 'NONE', #12072, #8085, #1072 ) ;
#3379=CARTESIAN_POINT ( 'NONE',  ( 48.49999999999995737, 90.00000000000000000, -8.000000000000000000 ) ) ;
#3395=ORIENTED_EDGE ( 'NONE', *, *, #8879, .T. ) ;
#3417=( NAMED_UNIT ( * ) PLANE_ANGLE_UNIT ( ) SI_UNIT ( $, .RADIAN. ) );
#3423=( GEOMETRIC_REPRESENTATION_CONTEXT ( 3 ) GLOBAL_UNCERTAINTY_ASSIGNED_CONTEXT ( ( #8007 ) ) GLOBAL_UNIT_ASSIGNED_CONTEXT ( ( #7207, #3417, #11193 ) ) REPRESENTATION_CONTEXT ( 'NONE', 'WORKASPACE' ) );
#3432=EDGE_CURVE ( 'NONE', #1735, #485, #8230, .T. ) ;
#3436=FACE_OUTER_BOUND ( 'NONE', #9725, .T. ) ;
#3439=DIRECTION ( 'NONE',  ( -0.000000000000000000, -0.000000000000000000, 1.000000000000000000 ) ) ;
#3443=EDGE_CURVE ( 'NONE', #1735, #9892, #1289, .T. ) ;
#3449=ORIENTED_EDGE ( 'NONE', *, *, #12633, .F. ) ;
#3469=VECTOR ( 'NONE', #12282, 1000.000000000000000 ) ;
#3488=LINE ( 'NONE', #3871, #11383 ) ;
#3497=EDGE_CURVE ( 'NONE', #8511, #2940, #3060, .T. ) ;
#3501=DIRECTION ( 'NONE',  ( 1.000000000000000000, 0.000000000000000000, 0.000000000000000000 ) ) ;
#3507=CARTESIAN_POINT ( 'NONE',  ( 35.00000000000000000, 90.00000000000000000, -3.799999999999999822 ) ) ;
#3515=AXIS2_PLACEMENT_3D ( 'NONE', #10372, #675, #8547 ) ;
#3520=DIRECTION ( 'NONE',  ( -0.3262398754384822630, 0.9452870165584014162, 0.000000000000000000 ) ) ;
#3524=VERTEX_POINT ( 'NONE', #5343 ) ;
#3532=EDGE_CURVE ( 'NONE', #485, #11942, #6179, .T. ) ;
#3533=AXIS2_PLACEMENT_3D ( 'NONE', #6458, #2352, #4506 ) ;
#3536=CARTESIAN_POINT ( 'NONE',  ( 34.25000000000000000, 93.26496554346289258, -3.799999999999999822 ) ) ;
#3560=DIRECTION ( 'NONE',  ( 1.000000000000000000, 0.000000000000000000, 0.000000000000000000 ) ) ;
#3565=EDGE_CURVE ( 'NONE', #2419, #2737, #11624, .T. ) ;
#3568=LINE ( 'NONE', #2580, #8461 ) ;
#3572=CARTESIAN_POINT ( 'NONE',  ( 31.96709571323326671, 88.25314809233525182, -3.799999999999999378 ) ) ;
#3582=DIRECTION ( 'NONE',  ( 0.8958148394926558344, 0.4444274669107966536, 4.977592430910269431E-17 ) ) ;
#3590=CARTESIAN_POINT ( 'NONE',  ( 48.49999999999995737, 90.00000000000000000, -10.00000000000000178 ) ) ;
#3595=VECTOR ( 'NONE', #9157, 1000.000000000000000 ) ;
#3600=DIRECTION ( 'NONE',  ( 0.000000000000000000, -0.000000000000000000, 1.000000000000000000 ) ) ;
#3607=EDGE_CURVE ( 'NONE', #8571, #7199, #9322, .T. ) ;
#3613=CARTESIAN_POINT ( 'NONE',  ( 35.00000000000000000, 90.00000000000000000, -8.000000000000000000 ) ) ;
#3619=ORIENTED_EDGE ( 'NONE', *, *, #7084, .F. ) ;
#3627=CARTESIAN_POINT ( 'NONE',  ( 35.00000000000000000, 90.00000000000000000, 4.800000000000000711 ) ) ;
#3630=CARTESIAN_POINT ( 'NONE',  ( 31.86869970978804290, 88.80942934165229019, 4.800000000000000711 ) ) ;
#3633=DIRECTION ( 'NONE',  ( 0.2967717757331703732, -0.9549484348006340717, -0.000000000000000000 ) ) ;
#3638=CARTESIAN_POINT ( 'NONE',  ( 35.00000000000000000, 90.00000000000000000, -3.000000000000000888 ) ) ;
#3660=EDGE_CURVE ( 'NONE', #7199, #8571, #6601, .T. ) ;
#3664=VECTOR ( 'NONE', #3439, 1000.000000000000000 ) ;
#3673=ORIENTED_EDGE ( 'NONE', *, *, #931, .F. ) ;
#3676=CIRCLE ( 'NONE', #5753, 1.599999999999986766 ) ;
#3677=EDGE_LOOP ( 'NONE', ( #12034, #1914, #1567, #5850 ) ) ;
#3683=DIRECTION ( 'NONE',  ( -1.000000000000000000, 0.000000000000000000, 0.000000000000000000 ) ) ;
#3707=ORIENTED_EDGE ( 'NONE', *, *, #8684, .F. ) ;
#3711=CARTESIAN_POINT ( 'NONE',  ( 21.49999999999998579, 94.00000000000000000, -10.00000000000000000 ) ) ;
#3728=ORIENTED_EDGE ( 'NONE', *, *, #8075, .T. ) ;
#3732=EDGE_LOOP ( 'NONE', ( #8175, #2147, #11196, #6726, #10411, #4835 ) ) ;
#3738=AXIS2_PLACEMENT_3D ( 'NONE', #11773, #10793, #12635 ) ;
#3742=ORIENTED_EDGE ( 'NONE', *, *, #9802, .T. ) ;
#3745=CARTESIAN_POINT ( 'NONE',  ( 35.00000000000000000, 90.00000000000000000, 4.800000000000000711 ) ) ;
#3747=VERTEX_POINT ( 'NONE', #2796 ) ;
#3749=ORIENTED_EDGE ( 'NONE', *, *, #9088, .T. ) ;
#3797=ORIENTED_EDGE ( 'NONE', *, *, #10741, .F. ) ;
#3803=FACE_OUTER_BOUND ( 'NONE', #4909, .T. ) ;
#3805=ORIENTED_EDGE ( 'NONE', *, *, #938, .F. ) ;
#3808=CARTESIAN_POINT ( 'NONE',  ( 48.49999999999995737, 90.00000000000000000, -10.00000000000000000 ) ) ;
#3838=CARTESIAN_POINT ( 'NONE',  ( 52.49999999999996447, 86.00000000000000000, -8.000000000000000000 ) ) ;
#3854=DIRECTION ( 'NONE',  ( -0.000000000000000000, -0.000000000000000000, -1.000000000000000000 ) ) ;
#3866=CARTESIAN_POINT ( 'NONE',  ( 52.49999999999996447, 86.00000000000000000, -10.00000000000000000 ) ) ;
#3869=AXIS2_PLACEMENT_3D ( 'NONE', #4414, #8404, #2454 ) ;
#3871=CARTESIAN_POINT ( 'NONE',  ( 31.86464806177570352, 88.44450386581220869, 6.000000000000000000 ) ) ;
#3883=CARTESIAN_POINT ( 'NONE',  ( 32.09707732552327286, 88.32801317409231956, -3.000000000000000000 ) ) ;
#3887=ORIENTED_EDGE ( 'NONE', *, *, #8474, .F. ) ;
#3904=EDGE_CURVE ( 'NONE', #4989, #8980, #10370, .T. ) ;
#3907=DIRECTION ( 'NONE',  ( 0.000000000000000000, 0.000000000000000000, 1.000000000000000000 ) ) ;
#3918=ADVANCED_FACE ( 'NONE', ( #9646 ), #5654, .T. ) ;
#3923=CARTESIAN_POINT ( 'NONE',  ( 35.00000000000000000, 90.00000000000000000, -18.00000000000000355 ) ) ;
#3925=EDGE_CURVE ( 'NONE', #11880, #5406, #11834, .T. ) ;
#3941=AXIS2_PLACEMENT_3D ( 'NONE', #1817, #7963, #5073 ) ;
#3952=DIRECTION ( 'NONE',  ( -0.000000000000000000, 0.000000000000000000, -1.000000000000000000 ) ) ;
#3953=CARTESIAN_POINT ( 'NONE',  ( 52.49999999999996447, 90.00000000000000000, -10.00000000000000000 ) ) ;
#3957=VERTEX_POINT ( 'NONE', #10568 ) ;
#3961=AXIS2_PLACEMENT_3D ( 'NONE', #10136, #7132, #1371 ) ;
#3968=CARTESIAN_POINT ( 'NONE',  ( 25.83484861008832567, 94.00000000000000000, -10.00000000000000000 ) ) ;
#3974=AXIS2_PLACEMENT_3D ( 'NONE', #3745, #10730, #1774 ) ;
#4001=DIRECTION ( 'NONE',  ( -0.000000000000000000, 0.000000000000000000, -1.000000000000000000 ) ) ;
#4022=LINE ( 'NONE', #7086, #4826 ) ;
#4031=CARTESIAN_POINT ( 'NONE',  ( 35.00000000000000000, 90.00000000000000000, -8.000000000000000000 ) ) ;
#4036=CIRCLE ( 'NONE', #6104, 3.500000000000003109 ) ;
#4038=EDGE_LOOP ( 'NONE', ( #12074, #5887, #12813, #3395 ) ) ;
#4046=EDGE_CURVE ( 'NONE', #4989, #681, #7284, .T. ) ;
#4050=EDGE_CURVE ( 'NONE', #408, #2666, #70, .T. ) ;
#4051=EDGE_LOOP ( 'NONE', ( #5358, #3887, #3728, #5402 ) ) ;
#4090=AXIS2_PLACEMENT_3D ( 'NONE', #6512, #6448, #6576 ) ;
#4096=CARTESIAN_POINT ( 'NONE',  ( 33.90709641728108892, 93.16671150547063007, 4.800000000000000711 ) ) ;
#4114=ORIENTED_EDGE ( 'NONE', *, *, #8856, .T. ) ;
#4120=EDGE_CURVE ( 'NONE', #5822, #6093, #11330, .T. ) ;
#4130=VERTEX_POINT ( 'NONE', #10420 ) ;
#4136=AXIS2_PLACEMENT_3D ( 'NONE', #7557, #8609, #9648 ) ;
#4146=ORIENTED_EDGE ( 'NONE', *, *, #2335, .T. ) ;
#4149=CYLINDRICAL_SURFACE ( 'NONE', #10258, 4.000000000000000000 ) ;
#4150=CARTESIAN_POINT ( 'NONE',  ( 31.72849223410691266, 88.75612020769642641, 6.000000000000000000 ) ) ;
#4155=CARTESIAN_POINT ( 'NONE',  ( 35.00000000000000000, 90.00000000000000000, 6.000000000000000000 ) ) ;
#4194=VERTEX_POINT ( 'NONE', #9693 ) ;
#4196=PLANE ( 'NONE',  #9164 ) ;
#4197=ORIENTED_EDGE ( 'NONE', *, *, #12920, .F. ) ;
#4202=DIRECTION ( 'NONE',  ( 0.9347165045408830641, 0.3553942263724511608, 0.000000000000000000 ) ) ;
#4204=DIRECTION ( 'NONE',  ( 0.000000000000000000, -0.000000000000000000, 1.000000000000000000 ) ) ;
#4208=ORIENTED_EDGE ( 'NONE', *, *, #3432, .F. ) ;
#4227=CARTESIAN_POINT ( 'NONE',  ( 35.75000000000000711, 93.41869858279433458, 6.000000000000000000 ) ) ;
#4229=CARTESIAN_POINT ( 'NONE',  ( 31.80092274341787828, 89.00581455129388075, 4.800000000000000711 ) ) ;
#4231=EDGE_LOOP ( 'NONE', ( #2622, #11507 ) ) ;
#4240=UNCERTAINTY_MEASURE_WITH_UNIT (LENGTH_MEASURE( 1.000000000000000082E-05 ), #9677, 'distance_accuracy_value', 'NONE');
#4244=VERTEX_POINT ( 'NONE', #12650 ) ;
#4247=EDGE_LOOP ( 'NONE', ( #6545, #8623, #5310, #11924, #6213 ) ) ;
#4269=DIRECTION ( 'NONE',  ( -0.000000000000000000, -0.000000000000000000, -1.000000000000000000 ) ) ;
#4290=DIRECTION ( 'NONE',  ( 1.000000000000000000, 0.000000000000000000, 0.000000000000000000 ) ) ;
#4298=FACE_OUTER_BOUND ( 'NONE', #11649, .T. ) ;
#4299=ORIENTED_EDGE ( 'NONE', *, *, #11783, .T. ) ;
#4311=AXIS2_PLACEMENT_3D ( 'NONE', #2971, #12782, #993 ) ;
#4322=ORIENTED_EDGE ( 'NONE', *, *, #12239, .F. ) ;
#4330=SHAPE_REPRESENTATION_RELATIONSHIP ( 'NONE' , 'NONE' ,  #5582, #8095 ) ;
#4337=EDGE_LOOP ( 'NONE', ( #10919, #2407 ) ) ;
#4351=DIRECTION ( 'NONE',  ( 0.000000000000000000, 0.000000000000000000, -1.000000000000000000 ) ) ;
#4375=ORIENTED_EDGE ( 'NONE', *, *, #2075, .T. ) ;
#4387=ORIENTED_EDGE ( 'NONE', *, *, #4599, .F. ) ;
#4394=FACE_BOUND ( 'NONE', #10586, .T. ) ;
#4402=VECTOR ( 'NONE', #6368, 1000.000000000000000 ) ;
#4410=CARTESIAN_POINT ( 'NONE',  ( 35.00000000000000000, 90.00000000000000000, -18.00000000000000355 ) ) ;
#4414=CARTESIAN_POINT ( 'NONE',  ( 35.00000000000000000, 90.00000000000000000, 4.000000000000000000 ) ) ;
#4415=DIRECTION ( 'NONE',  ( 1.000000000000000000, 0.000000000000000000, 0.000000000000000000 ) ) ;
#4422=CARTESIAN_POINT ( 'NONE',  ( 34.25000000000000000, 92.49999999999998579, -8.000000000000000000 ) ) ;
#4430=ORIENTED_EDGE ( 'NONE', *, *, #1875, .F. ) ;
#4439=EDGE_LOOP ( 'NONE', ( #10915, #7711, #8975, #2361 ) ) ;
#4447=VERTEX_POINT ( 'NONE', #9662 ) ;
#4455=FACE_OUTER_BOUND ( 'NONE', #12847, .T. ) ;
#4458=EDGE_CURVE ( 'NONE', #4244, #370, #11851, .T. ) ;
#4486=PLANE ( 'NONE',  #5373 ) ;
#4491=CIRCLE ( 'NONE', #3033, 4.000000000000000000 ) ;
#4492=DIRECTION ( 'NONE',  ( -0.000000000000000000, -0.000000000000000000, -1.000000000000000000 ) ) ;
#4496=AXIS2_PLACEMENT_3D ( 'NONE', #1220, #5212, #9202 ) ;
#4506=DIRECTION ( 'NONE',  ( 0.4719909656437444867, -0.8816033849473842166, 0.000000000000000000 ) ) ;
#4507=CIRCLE ( 'NONE', #12855, 1.599999999999990319 ) ;
#4510=AXIS2_PLACEMENT_3D ( 'NONE', #8551, #12402, #5838 ) ;
#4515=CARTESIAN_POINT ( 'NONE',  ( 48.49999999999995737, 94.00000000000000000, -10.00000000000000000 ) ) ;
#4525=LINE ( 'NONE', #8448, #4564 ) ;
#4543=DIRECTION ( 'NONE',  ( 0.000000000000000000, 0.000000000000000000, -1.000000000000000000 ) ) ;
#4546=DIRECTION ( 'NONE',  ( -0.000000000000000000, -0.000000000000000000, -1.000000000000000000 ) ) ;
#4560=ORIENTED_EDGE ( 'NONE', *, *, #531, .T. ) ;
#4564=VECTOR ( 'NONE', #11516, 1000.000000000000000 ) ;
#4577=DIRECTION ( 'NONE',  ( -5.624500927088228034E-17, 1.370729058197317775E-18, 1.000000000000000000 ) ) ;
#4581=ORIENTED_EDGE ( 'NONE', *, *, #6194, .T. ) ;
#4588=FACE_BOUND ( 'NONE', #11738, .T. ) ;
#4599=EDGE_CURVE ( 'NONE', #5406, #12152, #12929, .T. ) ;
#4600=ORIENTED_EDGE ( 'NONE', *, *, #3904, .T. ) ;
#4608=VECTOR ( 'NONE', #1274, 1000.000000000000227 ) ;
#4620=DIRECTION ( 'NONE',  ( 0.000000000000000000, -0.000000000000000000, 1.000000000000000000 ) ) ;
#4631=DIRECTION ( 'NONE',  ( -0.000000000000000000, -0.000000000000000000, -1.000000000000000000 ) ) ;
#4638=CARTESIAN_POINT ( 'NONE',  ( 46.89999999999997016, 90.00000000000000000, -8.000000000000000000 ) ) ;
#4640=CARTESIAN_POINT ( 'NONE',  ( 21.49999999999998579, 86.00000000000000000, -8.000000000000000000 ) ) ;
#4650=EDGE_LOOP ( 'NONE', ( #6615, #2415, #9300, #4322 ) ) ;
#4654=DIRECTION ( 'NONE',  ( -0.000000000000000000, -0.000000000000000000, 1.000000000000000000 ) ) ;
#4664=VECTOR ( 'NONE', #2010, 1000.000000000000000 ) ;
#4681=ADVANCED_FACE ( 'NONE', ( #4298 ), #5267, .F. ) ;
#4695=AXIS2_PLACEMENT_3D ( 'NONE', #10167, #2064, #341 ) ;
#4697=VERTEX_POINT ( 'NONE', #1211 ) ;
#4753=CARTESIAN_POINT ( 'NONE',  ( 25.83484861008832567, 86.00000000000000000, -8.000000000000000000 ) ) ;
#4783=VERTEX_POINT ( 'NONE', #7299 ) ;
#4791=CYLINDRICAL_SURFACE ( 'NONE', #3191, 3.349999999999995204 ) ;
#4792=VECTOR ( 'NONE', #12749, 1000.000000000000000 ) ;
#4798=DIRECTION ( 'NONE',  ( -0.000000000000000000, -0.000000000000000000, -1.000000000000000000 ) ) ;
#4802=AXIS2_PLACEMENT_3D ( 'NONE', #8774, #1968, #7919 ) ;
#4812=VECTOR ( 'NONE', #1020, 1000.000000000000000 ) ;
#4817=CIRCLE ( 'NONE', #839, 3.500000000000003109 ) ;
#4824=DIRECTION ( 'NONE',  ( 0.000000000000000000, 0.000000000000000000, 1.000000000000000000 ) ) ;
#4826=VECTOR ( 'NONE', #6097, 1000.000000000000000 ) ;
#4829=ADVANCED_FACE ( 'NONE', ( #6439, #10571 ), #4486, .F. ) ;
#4835=ORIENTED_EDGE ( 'NONE', *, *, #2335, .F. ) ;
#4841=CYLINDRICAL_SURFACE ( 'NONE', #879, 3.350000000000003642 ) ;
#4847=AXIS2_PLACEMENT_3D ( 'NONE', #7493, #7182, #12467 ) ;
#4848=CARTESIAN_POINT ( 'NONE',  ( 45.00000000000000711, 90.00000000000000000, -10.00000000000000000 ) ) ;
#4856=AXIS2_PLACEMENT_3D ( 'NONE', #9159, #185, #4202 ) ;
#4872=EDGE_CURVE ( 'NONE', #9364, #8511, #11010, .T. ) ;
#4873=EDGE_CURVE ( 'NONE', #294, #216, #2464, .T. ) ;
#4879=EDGE_CURVE ( 'NONE', #4783, #1668, #2887, .T. ) ;
#4886=DIRECTION ( 'NONE',  ( 1.000000000000000000, 0.000000000000000000, 0.000000000000000000 ) ) ;
#4889=DIRECTION ( 'NONE',  ( 1.000000000000000000, 0.000000000000000000, 0.000000000000000000 ) ) ;
#4903=EDGE_CURVE ( 'NONE', #7314, #6404, #12699, .T. ) ;
#4904=LINE ( 'NONE', #3866, #8629 ) ;
#4909=EDGE_LOOP ( 'NONE', ( #1363, #5983, #8882, #4197, #8934, #1950, #6009, #7083, #11297, #1572, #7471, #543 ) ) ;
#4933=AXIS2_PLACEMENT_3D ( 'NONE', #11800, #1988, #5965 ) ;
#4941=VECTOR ( 'NONE', #11268, 1000.000000000000000 ) ;
#4957=DIRECTION ( 'NONE',  ( 0.000000000000000000, -1.000000000000000000, 0.000000000000000000 ) ) ;
#4963=VERTEX_POINT ( 'NONE', #8731 ) ;
#4972=FACE_OUTER_BOUND ( 'NONE', #2548, .T. ) ;
#4987=PLANE ( 'NONE',  #8343 ) ;
#4989=VERTEX_POINT ( 'NONE', #6827 ) ;
#4990=CARTESIAN_POINT ( 'NONE',  ( 48.49999999999995737, 86.00000000000000000, -10.00000000000000000 ) ) ;
#4992=CIRCLE ( 'NONE', #1012, 3.500000000000003109 ) ;
#5004=CARTESIAN_POINT ( 'NONE',  ( 31.99902028769960438, 88.51116798584881451, -3.800000000000000266 ) ) ;
#5008=VECTOR ( 'NONE', #10116, 1000.000000000000000 ) ;
#5010=EDGE_LOOP ( 'NONE', ( #6873, #6864, #12485, #9083 ) ) ;
#5018=VECTOR ( 'NONE', #4543, 1000.000000000000000 ) ;
#5020=DIRECTION ( 'NONE',  ( 0.000000000000000000, 0.000000000000000000, -1.000000000000000000 ) ) ;
#5023=EDGE_CURVE ( 'NONE', #11514, #29, #980, .T. ) ;
#5042=FACE_OUTER_BOUND ( 'NONE', #8316, .T. ) ;
#5056=LINE ( 'NONE', #8144, #12066 ) ;
#5058=CARTESIAN_POINT ( 'NONE',  ( 35.00000000000000000, 90.00000000000000000, -3.000000000000000000 ) ) ;
#5063=EDGE_CURVE ( 'NONE', #681, #6762, #869, .T. ) ;
#5073=DIRECTION ( 'NONE',  ( -1.000000000000000000, 0.000000000000000000, 0.000000000000000000 ) ) ;
#5082=EDGE_CURVE ( 'NONE', #5372, #237, #5056, .T. ) ;
#5087=DIRECTION ( 'NONE',  ( -0.000000000000000000, -0.000000000000000000, -1.000000000000000000 ) ) ;
#5089=VECTOR ( 'NONE', #10713, 1000.000000000000000 ) ;
#5090=ORIENTED_EDGE ( 'NONE', *, *, #10556, .F. ) ;
#5110=CIRCLE ( 'NONE', #83, 1.599999999999990319 ) ;
#5115=CARTESIAN_POINT ( 'NONE',  ( 35.00000000000000000, 90.00000000000000000, -3.799999999999999822 ) ) ;
#5116=ORIENTED_EDGE ( 'NONE', *, *, #12486, .T. ) ;
#5120=VERTEX_POINT ( 'NONE', #10162 ) ;
#5122=DIRECTION ( 'NONE',  ( 0.000000000000000000, -1.000000000000000000, -0.000000000000000000 ) ) ;
#5123=AXIS2_PLACEMENT_3D ( 'NONE', #8096, #7905, #12084 ) ;
#5133=DIRECTION ( 'NONE',  ( -1.000000000000000000, 0.000000000000000000, 0.000000000000000000 ) ) ;
#5144=DIRECTION ( 'NONE',  ( -0.000000000000000000, -0.000000000000000000, 1.000000000000000000 ) ) ;
#5166=DIRECTION ( 'NONE',  ( 0.000000000000000000, 0.000000000000000000, -1.000000000000000000 ) ) ;
#5171=PLANE ( 'NONE',  #4856 ) ;
#5175=ADVANCED_FACE ( 'NONE', ( #1128 ), #9179, .F. ) ;
#5192=AXIS2_PLACEMENT_3D ( 'NONE', #8044, #5087, #107 ) ;
#5195=CARTESIAN_POINT ( 'NONE',  ( 31.86869970978804290, 88.80942934165229019, 4.000000000000000000 ) ) ;
#5199=DIRECTION ( 'NONE',  ( 0.000000000000000000, 0.000000000000000000, -1.000000000000000000 ) ) ;
#5211=ORIENTED_EDGE ( 'NONE', *, *, #4872, .F. ) ;
#5212=DIRECTION ( 'NONE',  ( 0.000000000000000000, 0.000000000000000000, -1.000000000000000000 ) ) ;
#5221=CARTESIAN_POINT ( 'NONE',  ( 35.00000000000000000, 90.00000000000000000, -3.799999999999999378 ) ) ;
#5234=DIRECTION ( 'NONE',  ( 0.4719909656437444867, -0.8816033849473842166, 0.000000000000000000 ) ) ;
#5240=CARTESIAN_POINT ( 'NONE',  ( 31.80092274341787828, 89.00581455129388075, 4.000000000000000000 ) ) ;
#5259=DIRECTION ( 'NONE',  ( -1.000000000000000000, 0.000000000000000000, 0.000000000000000000 ) ) ;
#5267=CYLINDRICAL_SURFACE ( 'NONE', #7465, 1.599999999999990319 ) ;
#5289=DIRECTION ( 'NONE',  ( 0.000000000000000000, 0.000000000000000000, 1.000000000000000000 ) ) ;
#5291=ORIENTED_EDGE ( 'NONE', *, *, #9934, .F. ) ;
#5310=ORIENTED_EDGE ( 'NONE', *, *, #3228, .T. ) ;
#5313=PRODUCT ( 'motor', 'motor', '', ( #1169 ) ) ;
#5323=LINE ( 'NONE', #11212, #6059 ) ;
#5343=CARTESIAN_POINT ( 'NONE',  ( 25.83484861008832567, 86.00000000000000000, -10.00000000000000000 ) ) ;
#5344=ORIENTED_EDGE ( 'NONE', *, *, #10071, .T. ) ;
#5350=CARTESIAN_POINT ( 'NONE',  ( 35.75000000000000711, 93.26496554346289258, -3.000000000000000000 ) ) ;
#5351=ORIENTED_EDGE ( 'NONE', *, *, #5023, .T. ) ;
#5358=ORIENTED_EDGE ( 'NONE', *, *, #4873, .F. ) ;
#5361=CARTESIAN_POINT ( 'NONE',  ( 38.50000000000000711, 90.00000000000000000, -3.799999999999999378 ) ) ;
#5366=ADVANCED_FACE ( 'NONE', ( #5042 ), #9228, .T. ) ;
#5372=VERTEX_POINT ( 'NONE', #11119 ) ;
#5373=AXIS2_PLACEMENT_3D ( 'NONE', #10631, #4620, #8481 ) ;
#5383=CARTESIAN_POINT ( 'NONE',  ( 21.49999999999998579, 90.00000000000000000, -10.00000000000000000 ) ) ;
#5390=VECTOR ( 'NONE', #9682, 1000.000000000000000 ) ;
#5392=EDGE_LOOP ( 'NONE', ( #12639, #10067, #12807, #3297 ) ) ;
#5398=CIRCLE ( 'NONE', #7076, 3.350000000000003642 ) ;
#5400=DIRECTION ( 'NONE',  ( -5.624500927088228034E-17, 1.370729058197317775E-18, 1.000000000000000000 ) ) ;
#5402=ORIENTED_EDGE ( 'NONE', *, *, #8986, .F. ) ;
#5405=AXIS2_PLACEMENT_3D ( 'NONE', #2808, #3854, #7710 ) ;
#5406=VERTEX_POINT ( 'NONE', #3094 ) ;
#5423=CARTESIAN_POINT ( 'NONE',  ( 35.00000000000000000, 90.00000000000000000, -3.000000000000000000 ) ) ;
#5429=CARTESIAN_POINT ( 'NONE',  ( 35.00000000000000000, 90.00000000000000000, 4.800000000000000711 ) ) ;
#5430=SURFACE_STYLE_USAGE ( .BOTH. , #11317 ) ;
#5434=EDGE_CURVE ( 'NONE', #252, #7199, #1180, .T. ) ;
#5445=FACE_OUTER_BOUND ( 'NONE', #5555, .T. ) ;
#5453=CARTESIAN_POINT ( 'NONE',  ( 31.86869970978804290, 88.80942934165229019, 4.000000000000000000 ) ) ;
#5469=DIRECTION ( 'NONE',  ( 0.000000000000000000, -0.000000000000000000, 1.000000000000000000 ) ) ;
#5479=VECTOR ( 'NONE', #2244, 1000.000000000000000 ) ;
#5486=ORIENTED_EDGE ( 'NONE', *, *, #5565, .T. ) ;
#5490=ORIENTED_EDGE ( 'NONE', *, *, #5990, .F. ) ;
#5493=CARTESIAN_POINT ( 'NONE',  ( 34.25000000000000000, 92.49999999999998579, 6.000000000000000000 ) ) ;
#5511=EDGE_CURVE ( 'NONE', #6093, #7515, #12574, .T. ) ;
#5518=DIRECTION ( 'NONE',  ( -0.000000000000000000, -0.000000000000000000, 1.000000000000000000 ) ) ;
#5521=CARTESIAN_POINT ( 'NONE',  ( 35.00000000000000000, 90.00000000000000000, 6.000000000000000000 ) ) ;
#5524=DIRECTION ( 'NONE',  ( 0.000000000000000000, 0.000000000000000000, -1.000000000000000000 ) ) ;
#5536=CIRCLE ( 'NONE', #10767, 3.500000000000003109 ) ;
#5547=DIRECTION ( 'NONE',  ( 0.4719909656437444867, -0.8816033849473842166, 0.000000000000000000 ) ) ;
#5555=EDGE_LOOP ( 'NONE', ( #3274, #12408, #1448, #10203, #1381, #11819, #1222, #3673 ) ) ;
#5565=EDGE_CURVE ( 'NONE', #8709, #9125, #4525, .T. ) ;
#5573=ORIENTED_EDGE ( 'NONE', *, *, #10170, .T. ) ;
#5579=EDGE_CURVE ( 'NONE', #2666, #681, #2680, .T. ) ;
#5582=SHAPE_REPRESENTATION ( 'motor', ( #5704 ), #898 ) ;
#5588=ADVANCED_FACE ( 'NONE', ( #12506, #4588, #4394, #2500 ), #8582, .F. ) ;
#5594=ORIENTED_EDGE ( 'NONE', *, *, #12195, .T. ) ;
#5601=FACE_OUTER_BOUND ( 'NONE', #5010, .T. ) ;
#5619=DIRECTION ( 'NONE',  ( 0.000000000000000000, 0.000000000000000000, -1.000000000000000000 ) ) ;
#5625=VECTOR ( 'NONE', #1816, 1000.000000000000000 ) ;
#5628=EDGE_CURVE ( 'NONE', #1353, #9660, #785, .T. ) ;
#5649=CARTESIAN_POINT ( 'NONE',  ( 31.80092274341787828, 89.00581455129388075, 4.800000000000000711 ) ) ;
#5651=CARTESIAN_POINT ( 'NONE',  ( 35.75000000000000711, 93.26496554346289258, 4.800000000000000711 ) ) ;
#5654=PLANE ( 'NONE',  #11416 ) ;
#5667=EDGE_CURVE ( 'NONE', #12821, #6093, #9811, .T. ) ;
#5683=ORIENTED_EDGE ( 'NONE', *, *, #5749, .F. ) ;
#5687=ORIENTED_EDGE ( 'NONE', *, *, #11376, .F. ) ;
#5694=LINE ( 'NONE', #840, #5390 ) ;
#5696=ORIENTED_EDGE ( 'NONE', *, *, #938, .T. ) ;
#5698=ORIENTED_EDGE ( 'NONE', *, *, #2269, .F. ) ;
#5699=EDGE_CURVE ( 'NONE', #10536, #7597, #5694, .T. ) ;
#5704=AXIS2_PLACEMENT_3D ( 'NONE', #8997, #4824, #4886 ) ;
#5712=ADVANCED_FACE ( 'NONE', ( #11710 ), #12889, .T. ) ;
#5735=CARTESIAN_POINT ( 'NONE',  ( 34.25000000000000000, 92.49999999999998579, -8.000000000000000000 ) ) ;
#5746=CYLINDRICAL_SURFACE ( 'NONE', #11696, 10.00000000000000178 ) ;
#5749=EDGE_CURVE ( 'NONE', #6072, #8571, #2758, .T. ) ;
#5753=AXIS2_PLACEMENT_3D ( 'NONE', #6120, #10115, #7307 ) ;
#5756=DIRECTION ( 'NONE',  ( 5.624500927088228034E-17, -1.370729058197317775E-18, -1.000000000000000000 ) ) ;
#5758=ADVANCED_FACE ( 'NONE', ( #3803 ), #7782, .F. ) ;
#5761=ORIENTED_EDGE ( 'NONE', *, *, #5082, .T. ) ;
#5776=DIRECTION ( 'NONE',  ( 0.000000000000000000, -0.000000000000000000, 1.000000000000000000 ) ) ;
#5781=CARTESIAN_POINT ( 'NONE',  ( 35.75000000000000711, 93.41869858279433458, 4.800000000000000711 ) ) ;
#5783=VERTEX_POINT ( 'NONE', #3077 ) ;
#5785=CARTESIAN_POINT ( 'NONE',  ( 21.49999999999998579, 90.00000000000000000, -8.000000000000000000 ) ) ;
#5801=EDGE_CURVE ( 'NONE', #2940, #2177, #10124, .T. ) ;
#5818=VECTOR ( 'NONE', #12618, 1000.000000000000000 ) ;
#5822=VERTEX_POINT ( 'NONE', #10975 ) ;
#5838=DIRECTION ( 'NONE',  ( 1.000000000000000000, 0.000000000000000000, 0.000000000000000000 ) ) ;
#5841=DIRECTION ( 'NONE',  ( -0.3262398754384822630, 0.9452870165584014162, 0.000000000000000000 ) ) ;
#5843=AXIS2_PLACEMENT_3D ( 'NONE', #8898, #5946, #6868 ) ;
#5850=ORIENTED_EDGE ( 'NONE', *, *, #3565, .F. ) ;
#5854=DIRECTION ( 'NONE',  ( 0.000000000000000000, -1.000000000000000000, 0.000000000000000000 ) ) ;
#5861=ORIENTED_EDGE ( 'NONE', *, *, #11783, .F. ) ;
#5872=DIRECTION ( 'NONE',  ( -0.000000000000000000, -0.000000000000000000, 1.000000000000000000 ) ) ;
#5878=CARTESIAN_POINT ( 'NONE',  ( 34.25000000000000000, 92.49999999999998579, -9.802775637731997449 ) ) ;
#5880=ORIENTED_EDGE ( 'NONE', *, *, #4458, .F. ) ;
#5887=ORIENTED_EDGE ( 'NONE', *, *, #1625, .F. ) ;
#5901=PLANE ( 'NONE',  #8644 ) ;
#5911=EDGE_CURVE ( 'NONE', #7597, #12207, #7278, .T. ) ;
#5926=EDGE_LOOP ( 'NONE', ( #6440, #5351, #10447, #4430, #1630, #1955, #12233, #6487, #12489, #6126 ) ) ;
#5937=VERTEX_POINT ( 'NONE', #5350 ) ;
#5940=ADVANCED_FACE ( 'NONE', ( #565 ), #7316, .T. ) ;
#5946=DIRECTION ( 'NONE',  ( -0.000000000000000000, -0.000000000000000000, -1.000000000000000000 ) ) ;
#5947=ORIENTED_EDGE ( 'NONE', *, *, #8951, .T. ) ;
#5950=ORIENTED_EDGE ( 'NONE', *, *, #5579, .T. ) ;
#5957=AXIS2_PLACEMENT_3D ( 'NONE', #4031, #2792, #7818 ) ;
#5962=DIRECTION ( 'NONE',  ( -0.000000000000000000, -0.000000000000000000, 1.000000000000000000 ) ) ;
#5965=DIRECTION ( 'NONE',  ( 1.000000000000000000, 0.000000000000000000, 0.000000000000000000 ) ) ;
#5972=AXIS2_PLACEMENT_3D ( 'NONE', #2346, #1223, #9205 ) ;
#5981=CARTESIAN_POINT ( 'NONE',  ( 35.00000000000000000, 90.00000000000000000, -18.00000000000000355 ) ) ;
#5983=ORIENTED_EDGE ( 'NONE', *, *, #8684, .T. ) ;
#5987=DIRECTION ( 'NONE',  ( -5.624500927088228034E-17, 1.370729058197317775E-18, 1.000000000000000000 ) ) ;
#5990=EDGE_CURVE ( 'NONE', #10917, #2123, #3278, .T. ) ;
#5991=DIRECTION ( 'NONE',  ( 0.000000000000000000, -0.000000000000000000, 1.000000000000000000 ) ) ;
#6007=EDGE_LOOP ( 'NONE', ( #1026, #10465, #2428, #11084 ) ) ;
#6009=ORIENTED_EDGE ( 'NONE', *, *, #10530, .F. ) ;
#6046=LINE ( 'NONE', #2005, #10663 ) ;
#6057=CIRCLE ( 'NONE', #9054, 4.000000000000003553 ) ;
#6059=VECTOR ( 'NONE', #8341, 1000.000000000000000 ) ;
#6072=VERTEX_POINT ( 'NONE', #4638 ) ;
#6083=LINE ( 'NONE', #8236, #12145 ) ;
#6093=VERTEX_POINT ( 'NONE', #11630 ) ;
#6097=DIRECTION ( 'NONE',  ( -0.000000000000000000, -0.000000000000000000, -1.000000000000000000 ) ) ;
#6103=EDGE_CURVE ( 'NONE', #2940, #9627, #10647, .T. ) ;
#6104=AXIS2_PLACEMENT_3D ( 'NONE', #5221, #430, #11299 ) ;
#6106=FACE_OUTER_BOUND ( 'NONE', #4650, .T. ) ;
#6108=CARTESIAN_POINT ( 'NONE',  ( 25.83484861008832567, 86.00000000000000000, -18.00000000000000355 ) ) ;
#6109=CYLINDRICAL_SURFACE ( 'NONE', #624, 1.599999999999990319 ) ;
#6118=CARTESIAN_POINT ( 'NONE',  ( 31.50000000000000000, 90.00000000000000000, 6.000000000000000000 ) ) ;
#6120=CARTESIAN_POINT ( 'NONE',  ( 21.49999999999998579, 90.00000000000000000, -10.00000000000000178 ) ) ;
#6121=LINE ( 'NONE', #10185, #5008 ) ;
#6123=CIRCLE ( 'NONE', #7605, 10.00000000000000178 ) ;
#6126=ORIENTED_EDGE ( 'NONE', *, *, #10746, .F. ) ;
#6141=DIRECTION ( 'NONE',  ( 5.624500927088228034E-17, -1.370729058197317775E-18, -1.000000000000000000 ) ) ;
#6156=CIRCLE ( 'NONE', #5123, 3.500000000000003109 ) ;
#6165=UNCERTAINTY_MEASURE_WITH_UNIT (LENGTH_MEASURE( 1.000000000000000082E-05 ), #7994, 'distance_accuracy_value', 'NONE');
#6172=FACE_OUTER_BOUND ( 'NONE', #5392, .T. ) ;
#6179=CIRCLE ( 'NONE', #10150, 10.00000000000000178 ) ;
#6182=ADVANCED_FACE ( 'NONE', ( #6781 ), #11008, .F. ) ;
#6186=AXIS2_PLACEMENT_3D ( 'NONE', #3638, #11343, #2586 ) ;
#6187=CARTESIAN_POINT ( 'NONE',  ( 35.75000000000000711, 92.49999999999998579, 6.000000000000000000 ) ) ;
#6193=DIRECTION ( 'NONE',  ( -1.000000000000000000, 0.000000000000000000, 0.000000000000000000 ) ) ;
#6194=EDGE_CURVE ( 'NONE', #1830, #12152, #9606, .T. ) ;
#6213=ORIENTED_EDGE ( 'NONE', *, *, #917, .T. ) ;
#6239=CYLINDRICAL_SURFACE ( 'NONE', #600, 3.500000000000003109 ) ;
#6241=DIRECTION ( 'NONE',  ( 1.000000000000000000, 0.000000000000000000, 0.000000000000000000 ) ) ;
#6245=CARTESIAN_POINT ( 'NONE',  ( 44.16515138991168499, 86.00000000000000000, -8.000000000000000000 ) ) ;
#6249=ORIENTED_EDGE ( 'NONE', *, *, #7392, .F. ) ;
#6262=CARTESIAN_POINT ( 'NONE',  ( 21.49999999999998579, 94.00000000000000000, -10.00000000000000000 ) ) ;
#6266=CARTESIAN_POINT ( 'NONE',  ( 25.00000000000000000, 90.00000000000000000, -18.00000000000000355 ) ) ;
#6271=ADVANCED_FACE ( 'NONE', ( #7154 ), #6239, .T. ) ;
#6283=CARTESIAN_POINT ( 'NONE',  ( 35.00000000000000000, 90.00000000000000000, 4.800000000000000711 ) ) ;
#6284=ADVANCED_FACE ( 'NONE', ( #6172 ), #8207, .T. ) ;
#6291=ORIENTED_EDGE ( 'NONE', *, *, #4050, .F. ) ;
#6293=ORIENTED_EDGE ( 'NONE', *, *, #310, .F. ) ;
#6298=DIRECTION ( 'NONE',  ( 0.000000000000000000, 0.000000000000000000, 1.000000000000000000 ) ) ;
#6302=CARTESIAN_POINT ( 'NONE',  ( 23.09999999999997300, 90.00000000000000000, -8.000000000000000000 ) ) ;
#6305=DIRECTION ( 'NONE',  ( -0.000000000000000000, -0.000000000000000000, 1.000000000000000000 ) ) ;
#6308=LINE ( 'NONE', #1530, #10242 ) ;
#6319=DIRECTION ( 'NONE',  ( 1.000000000000000000, 0.000000000000000000, 0.000000000000000000 ) ) ;
#6322=VECTOR ( 'NONE', #1554, 1000.000000000000000 ) ;
#6329=VERTEX_POINT ( 'NONE', #9313 ) ;
#6331=LINE ( 'NONE', #1299, #12230 ) ;
#6352=ORIENTED_EDGE ( 'NONE', *, *, #1216, .F. ) ;
#6358=VECTOR ( 'NONE', #4492, 1000.000000000000000 ) ;
#6366=AXIS2_PLACEMENT_3D ( 'NONE', #9889, #5776, #8786 ) ;
#6368=DIRECTION ( 'NONE',  ( 1.000000000000000000, -0.000000000000000000, -0.000000000000000000 ) ) ;
#6376=VECTOR ( 'NONE', #3683, 1000.000000000000000 ) ;
#6391=VECTOR ( 'NONE', #9273, 1000.000000000000000 ) ;
#6395=ADVANCED_FACE ( 'NONE', ( #5445 ), #2577, .T. ) ;
#6404=VERTEX_POINT ( 'NONE', #9375 ) ;
#6405=DIRECTION ( 'NONE',  ( 1.000000000000000000, -0.000000000000000000, 0.000000000000000000 ) ) ;
#6431=CARTESIAN_POINT ( 'NONE',  ( 31.65768047819777919, 88.96129878493390208, 6.000000000000000000 ) ) ;
#6439=FACE_BOUND ( 'NONE', #4337, .T. ) ;
#6440=ORIENTED_EDGE ( 'NONE', *, *, #9934, .T. ) ;
#6443=LINE ( 'NONE', #11616, #914 ) ;
#6446=AXIS2_PLACEMENT_3D ( 'NONE', #9416, #8382, #8183 ) ;
#6448=DIRECTION ( 'NONE',  ( 0.4444274669107966536, -0.8958148394926558344, 2.622474642788943734E-17 ) ) ;
#6452=VERTEX_POINT ( 'NONE', #10423 ) ;
#6458=CARTESIAN_POINT ( 'NONE',  ( 35.00000000000000000, 90.00000000000000000, -3.799999999999999822 ) ) ;
#6473=ADVANCED_FACE ( 'NONE', ( #7263 ), #10205, .F. ) ;
#6476=CARTESIAN_POINT ( 'NONE',  ( 35.75000000000000711, 93.26496554346289258, 4.800000000000000711 ) ) ;
#6487=ORIENTED_EDGE ( 'NONE', *, *, #11483, .F. ) ;
#6497=LINE ( 'NONE', #11536, #7405 ) ;
#6503=LINE ( 'NONE', #4422, #10485 ) ;
#6506=ADVANCED_FACE ( 'NONE', ( #12366 ), #4196, .F. ) ;
#6509=LINE ( 'NONE', #10504, #12456 ) ;
#6512=CARTESIAN_POINT ( 'NONE',  ( 31.99902028769960438, 88.51116798584881451, -3.800000000000000266 ) ) ;
#6519=AXIS2_PLACEMENT_3D ( 'NONE', #2108, #6940, #7072 ) ;
#6521=ORIENTED_EDGE ( 'NONE', *, *, #7923, .T. ) ;
#6527=ORIENTED_EDGE ( 'NONE', *, *, #3532, .T. ) ;
#6536=EDGE_CURVE ( 'NONE', #5937, #12562, #5398, .T. ) ;
#6537=DIRECTION ( 'NONE',  ( 0.000000000000000000, 1.000000000000000000, 0.000000000000000000 ) ) ;
#6545=ORIENTED_EDGE ( 'NONE', *, *, #1625, .T. ) ;
#6547=MECHANICAL_DESIGN_GEOMETRIC_PRESENTATION_REPRESENTATION('',(#1959),#3423);
#6557=PRODUCT_DEFINITION_FORMATION_WITH_SPECIFIED_SOURCE ( 'ANY', '', #5313, .NOT_KNOWN. ) ;
#6560=DIRECTION ( 'NONE',  ( -0.000000000000000000, -0.000000000000000000, -1.000000000000000000 ) ) ;
#6561=CARTESIAN_POINT ( 'NONE',  ( 31.80092274341787828, 89.00581455129388075, 4.800000000000000711 ) ) ;
#6576=DIRECTION ( 'NONE',  ( 0.8958148394926558344, 0.4444274669107966536, 4.977592430910269431E-17 ) ) ;
#6577=EDGE_CURVE ( 'NONE', #7985, #5120, #8748, .T. ) ;
#6587=CIRCLE ( 'NONE', #5957, 10.00000000000000178 ) ;
#6592=CARTESIAN_POINT ( 'NONE',  ( 35.00000000000000000, 90.00000000000000000, -8.000000000000000000 ) ) ;
#6594=CARTESIAN_POINT ( 'NONE',  ( 35.00000000000000000, 90.00000000000000000, -18.00000000000000355 ) ) ;
#6601=CIRCLE ( 'NONE', #7856, 1.599999999999990319 ) ;
#6615=ORIENTED_EDGE ( 'NONE', *, *, #8639, .F. ) ;
#6634=DIRECTION ( 'NONE',  ( -0.000000000000000000, -0.000000000000000000, -1.000000000000000000 ) ) ;
#6653=AXIS2_PLACEMENT_3D ( 'NONE', #11334, #1392, #8145 ) ;
#6668=EDGE_LOOP ( 'NONE', ( #644, #2231, #6730, #12036 ) ) ;
#6692=CARTESIAN_POINT ( 'NONE',  ( 21.49999999999998579, 90.00000000000000000, -10.00000000000000000 ) ) ;
#6701=( NAMED_UNIT ( * ) PLANE_ANGLE_UNIT ( ) SI_UNIT ( $, .RADIAN. ) );
#6706=STYLED_ITEM('',(#13016),#11745);
#6726=ORIENTED_EDGE ( 'NONE', *, *, #19, .F. ) ;
#6729=( NAMED_UNIT ( * ) PLANE_ANGLE_UNIT ( ) SI_UNIT ( $, .RADIAN. ) );
#6730=ORIENTED_EDGE ( 'NONE', *, *, #12241, .T. ) ;
#6740=LINE ( 'NONE', #10733, #9885 ) ;
#6749=CYLINDRICAL_SURFACE ( 'NONE', #11612, 3.500000000000003109 ) ;
#6762=VERTEX_POINT ( 'NONE', #3630 ) ;
#6777=ORIENTED_EDGE ( 'NONE', *, *, #10093, .T. ) ;
#6781=FACE_OUTER_BOUND ( 'NONE', #3732, .T. ) ;
#6790=EDGE_LOOP ( 'NONE', ( #5594, #2674, #2739, #11064, #2910, #2103 ) ) ;
#6798=LINE ( 'NONE', #9013, #12379 ) ;
#6812=AXIS2_PLACEMENT_3D ( 'NONE', #3590, #4631, #11557 ) ;
#6827=CARTESIAN_POINT ( 'NONE',  ( 31.72849223410691266, 88.75612020769642641, 4.000000000000000000 ) ) ;
#6828=ORIENTED_EDGE ( 'NONE', *, *, #12589, .F. ) ;
#6862=DIRECTION ( 'NONE',  ( 0.4719909656437444867, -0.8816033849473842166, 0.000000000000000000 ) ) ;
#6864=ORIENTED_EDGE ( 'NONE', *, *, #6194, .F. ) ;
#6868=DIRECTION ( 'NONE',  ( -1.000000000000000000, 0.000000000000000000, 0.000000000000000000 ) ) ;
#6873=ORIENTED_EDGE ( 'NONE', *, *, #4599, .T. ) ;
#6896=VECTOR ( 'NONE', #4957, 1000.000000000000000 ) ;
#6924=CARTESIAN_POINT ( 'NONE',  ( 31.50000000000000000, 90.00000000000000000, -3.000000000000000888 ) ) ;
#6940=DIRECTION ( 'NONE',  ( 0.000000000000000000, 0.000000000000000000, -1.000000000000000000 ) ) ;
#6958=DIRECTION ( 'NONE',  ( -1.000000000000000000, 0.000000000000000000, 0.000000000000000000 ) ) ;
#6996=ADVANCED_FACE ( 'NONE', ( #11195, #8063 ), #10146, .F. ) ;
#6998=CARTESIAN_POINT ( 'NONE',  ( 35.00000000000000000, 90.00000000000000000, 6.000000000000000000 ) ) ;
#7014=VERTEX_POINT ( 'NONE', #2176 ) ;
#7020=ORIENTED_EDGE ( 'NONE', *, *, #1724, .F. ) ;
#7030=CARTESIAN_POINT ( 'NONE',  ( 31.72849223410691266, 88.75612020769642641, 4.800000000000000711 ) ) ;
#7032=DIRECTION ( 'NONE',  ( 1.000000000000000000, 0.000000000000000000, 0.000000000000000000 ) ) ;
#7033=ADVANCED_FACE ( 'NONE', ( #251 ), #7995, .T. ) ;
#7037=ORIENTED_EDGE ( 'NONE', *, *, #9057, .T. ) ;
#7054=ADVANCED_FACE ( 'NONE', ( #8969 ), #56, .F. ) ;
#7072=DIRECTION ( 'NONE',  ( -1.000000000000000000, 0.000000000000000000, 0.000000000000000000 ) ) ;
#7075=DIRECTION ( 'NONE',  ( -0.4991005450470686888, 0.8665440819333538602, -2.925971193658973835E-17 ) ) ;
#7076=AXIS2_PLACEMENT_3D ( 'NONE', #5423, #6141, #5234 ) ;
#7083=ORIENTED_EDGE ( 'NONE', *, *, #8075, .F. ) ;
#7084=EDGE_CURVE ( 'NONE', #1830, #12608, #1870, .T. ) ;
#7085=AXIS2_PLACEMENT_3D ( 'NONE', #3248, #3181, #4415 ) ;
#7086=CARTESIAN_POINT ( 'NONE',  ( 21.49999999999998579, 86.00000000000000000, -10.00000000000000000 ) ) ;
#7100=ORIENTED_EDGE ( 'NONE', *, *, #7619, .F. ) ;
#7122=DIRECTION ( 'NONE',  ( -0.8665440819333538602, -0.4991005450470686888, -4.805464830191153728E-17 ) ) ;
#7132=DIRECTION ( 'NONE',  ( 0.000000000000000000, 1.000000000000000000, 0.000000000000000000 ) ) ;
#7138=VECTOR ( 'NONE', #6537, 1000.000000000000000 ) ;
#7149=CARTESIAN_POINT ( 'NONE',  ( 34.25000000000000000, 92.49999999999998579, -3.000000000000000000 ) ) ;
#7151=ORIENTED_EDGE ( 'NONE', *, *, #867, .F. ) ;
#7154=FACE_OUTER_BOUND ( 'NONE', #7558, .T. ) ;
#7174=CARTESIAN_POINT ( 'NONE',  ( 45.00000000000000711, 90.00000000000000000, -18.00000000000000355 ) ) ;
#7182=DIRECTION ( 'NONE',  ( 0.000000000000000000, -0.000000000000000000, 1.000000000000000000 ) ) ;
#7199=VERTEX_POINT ( 'NONE', #7334 ) ;
#7204=CIRCLE ( 'NONE', #3869, 3.349999999999995204 ) ;
#7207=( LENGTH_UNIT ( ) NAMED_UNIT ( * ) SI_UNIT ( .MILLI., .METRE. ) );
#7212=AXIS2_PLACEMENT_3D ( 'NONE', #10381, #5144, #1414 ) ;
#7216=PLANE ( 'NONE',  #12188 ) ;
#7221=CARTESIAN_POINT ( 'NONE',  ( 52.49999999999996447, 94.00000000000000000, -10.00000000000000000 ) ) ;
#7222=AXIS2_PLACEMENT_3D ( 'NONE', #6692, #4546, #10687 ) ;
#7228=DIRECTION ( 'NONE',  ( 1.000000000000000000, 0.000000000000000000, 0.000000000000000000 ) ) ;
#7232=VECTOR ( 'NONE', #8299, 1000.000000000000000 ) ;
#7238=ORIENTED_EDGE ( 'NONE', *, *, #693, .F. ) ;
#7251=AXIS2_PLACEMENT_3D ( 'NONE', #12414, #1552, #1487 ) ;
#7257=AXIS2_PLACEMENT_3D ( 'NONE', #12535, #5524, #1405 ) ;
#7263=FACE_OUTER_BOUND ( 'NONE', #8698, .T. ) ;
#7267=LINE ( 'NONE', #8317, #3595 ) ;
#7278=CIRCLE ( 'NONE', #5192, 1.599999999999986766 ) ;
#7284=LINE ( 'NONE', #4150, #4941 ) ;
#7296=CARTESIAN_POINT ( 'NONE',  ( 52.49999999999996447, 94.00000000000000000, -8.000000000000000000 ) ) ;
#7299=CARTESIAN_POINT ( 'NONE',  ( 25.00000000000000000, 90.00000000000000000, -18.00000000000000355 ) ) ;
#7306=ORIENTED_EDGE ( 'NONE', *, *, #5565, .F. ) ;
#7307=DIRECTION ( 'NONE',  ( -1.000000000000000000, 0.000000000000000000, 0.000000000000000000 ) ) ;
#7314=VERTEX_POINT ( 'NONE', #9917 ) ;
#7316=CYLINDRICAL_SURFACE ( 'NONE', #3533, 3.350000000000003642 ) ;
#7334=CARTESIAN_POINT ( 'NONE',  ( 50.09999999999995168, 90.00000000000000000, -10.00000000000000178 ) ) ;
#7355=DIRECTION ( 'NONE',  ( -1.000000000000000000, 0.000000000000000000, 0.000000000000000000 ) ) ;
#7358=DIRECTION ( 'NONE',  ( 1.000000000000000000, 0.000000000000000000, 0.000000000000000000 ) ) ;
#7374=CARTESIAN_POINT ( 'NONE',  ( 35.00000000000000000, 90.00000000000000000, -10.00000000000000000 ) ) ;
#7388=ORIENTED_EDGE ( 'NONE', *, *, #4879, .T. ) ;
#7392=EDGE_CURVE ( 'NONE', #9125, #191, #11870, .T. ) ;
#7398=AXIS2_PLACEMENT_3D ( 'NONE', #1612, #12669, #8552 ) ;
#7405=VECTOR ( 'NONE', #2457, 1000.000000000000000 ) ;
#7417=AXIS2_PLACEMENT_3D ( 'NONE', #8147, #3179, #6241 ) ;
#7419=DIRECTION ( 'NONE',  ( 0.4719909656437442647, -0.8816033849473842166, 2.775557561595757269E-17 ) ) ;
#7420=DIRECTION ( 'NONE',  ( -1.000000000000000000, 0.000000000000000000, 0.000000000000000000 ) ) ;
#7422=CYLINDRICAL_SURFACE ( 'NONE', #7222, 1.599999999999990319 ) ;
#7434=VECTOR ( 'NONE', #6305, 1000.000000000000000 ) ;
#7436=PLANE ( 'NONE',  #7398 ) ;
#7447=EDGE_CURVE ( 'NONE', #6762, #8980, #1343, .T. ) ;
#7452=CARTESIAN_POINT ( 'NONE',  ( 35.75000000000000711, 93.26496554346289258, 4.000000000000000000 ) ) ;
#7465=AXIS2_PLACEMENT_3D ( 'NONE', #2207, #12273, #11149 ) ;
#7471=ORIENTED_EDGE ( 'NONE', *, *, #531, .F. ) ;
#7489=CARTESIAN_POINT ( 'NONE',  ( 48.49999999999995737, 90.00000000000000000, -10.00000000000000000 ) ) ;
#7490=DIRECTION ( 'NONE',  ( 0.000000000000000000, 0.000000000000000000, 1.000000000000000000 ) ) ;
#7493=CARTESIAN_POINT ( 'NONE',  ( 48.49999999999995737, 90.00000000000000000, -10.00000000000000000 ) ) ;
#7508=AXIS2_PLACEMENT_3D ( 'NONE', #10098, #9119, #4290 ) ;
#7515=VERTEX_POINT ( 'NONE', #6187 ) ;
#7535=CARTESIAN_POINT ( 'NONE',  ( 32.09707732552327286, 88.32801317409231956, -3.000000000000000000 ) ) ;
#7547=EDGE_CURVE ( 'NONE', #8908, #12207, #10307, .T. ) ;
#7550=CYLINDRICAL_SURFACE ( 'NONE', #1769, 3.349999999999995204 ) ;
#7556=CYLINDRICAL_SURFACE ( 'NONE', #4847, 4.000000000000003553 ) ;
#7557=CARTESIAN_POINT ( 'NONE',  ( 35.00000000000000000, 90.00000000000000000, -3.000000000000000888 ) ) ;
#7558=EDGE_LOOP ( 'NONE', ( #5687, #7688, #6521, #5761 ) ) ;
#7583=CARTESIAN_POINT ( 'NONE',  ( 31.50000000000000000, 90.00000000000000000, 4.000000000000000000 ) ) ;
#7597=VERTEX_POINT ( 'NONE', #2663 ) ;
#7605=AXIS2_PLACEMENT_3D ( 'NONE', #11758, #5991, #12805 ) ;
#7619=EDGE_CURVE ( 'NONE', #237, #9364, #6443, .T. ) ;
#7658=DIRECTION ( 'NONE',  ( -1.000000000000000000, 0.000000000000000000, 0.000000000000000000 ) ) ;
#7688=ORIENTED_EDGE ( 'NONE', *, *, #2653, .T. ) ;
#7710=DIRECTION ( 'NONE',  ( -1.000000000000000000, 0.000000000000000000, 0.000000000000000000 ) ) ;
#7711=ORIENTED_EDGE ( 'NONE', *, *, #1595, .T. ) ;
#7716=ORIENTED_EDGE ( 'NONE', *, *, #1875, .T. ) ;
#7721=CARTESIAN_POINT ( 'NONE',  ( 35.00000000000000000, 90.00000000000000000, -3.799999999999999822 ) ) ;
#7723=AXIS2_PLACEMENT_3D ( 'NONE', #3808, #4001, #9876 ) ;
#7725=ORIENTED_EDGE ( 'NONE', *, *, #9057, .F. ) ;
#7762=DIRECTION ( 'NONE',  ( 0.8958148394926558344, 0.4444274669107966536, 4.977592430910269431E-17 ) ) ;
#7770=ORIENTED_EDGE ( 'NONE', *, *, #9281, .F. ) ;
#7773=ORIENTED_EDGE ( 'NONE', *, *, #1503, .F. ) ;
#7782=PLANE ( 'NONE',  #3738 ) ;
#7795=CARTESIAN_POINT ( 'NONE',  ( 31.99902028769960438, 88.51116798584881451, -3.000000000000000000 ) ) ;
#7800=CARTESIAN_POINT ( 'NONE',  ( 21.49999999999998579, 90.00000000000000000, -10.00000000000000000 ) ) ;
#7818=DIRECTION ( 'NONE',  ( -1.000000000000000000, 0.000000000000000000, 0.000000000000000000 ) ) ;
#7837=VERTEX_POINT ( 'NONE', #10762 ) ;
#7843=CARTESIAN_POINT ( 'NONE',  ( 35.00000000000000000, 90.00000000000000000, 4.800000000000000711 ) ) ;
#7848=CARTESIAN_POINT ( 'NONE',  ( 35.00000000000000000, 90.00000000000000000, 4.000000000000000000 ) ) ;
#7856=AXIS2_PLACEMENT_3D ( 'NONE', #8619, #2604, #8495 ) ;
#7905=DIRECTION ( 'NONE',  ( 0.000000000000000000, 0.000000000000000000, -1.000000000000000000 ) ) ;
#7919=DIRECTION ( 'NONE',  ( -1.000000000000000000, 0.000000000000000000, 0.000000000000000000 ) ) ;
#7923=EDGE_CURVE ( 'NONE', #5783, #5372, #12844, .T. ) ;
#7928=LINE ( 'NONE', #3883, #9019 ) ;
#7950=VECTOR ( 'NONE', #9055, 1000.000000000000000 ) ;
#7955=CYLINDRICAL_SURFACE ( 'NONE', #3364, 3.500000000000003109 ) ;
#7963=DIRECTION ( 'NONE',  ( 0.000000000000000000, 0.000000000000000000, -1.000000000000000000 ) ) ;
#7977=CARTESIAN_POINT ( 'NONE',  ( 34.25000000000000000, 93.26496554346289258, -3.799999999999999822 ) ) ;
#7980=VERTEX_POINT ( 'NONE', #401 ) ;
#7981=( GEOMETRIC_REPRESENTATION_CONTEXT ( 3 ) GLOBAL_UNCERTAINTY_ASSIGNED_CONTEXT ( ( #4240 ) ) GLOBAL_UNIT_ASSIGNED_CONTEXT ( ( #9677, #6729, #9618 ) ) REPRESENTATION_CONTEXT ( 'NONE', 'WORKASPACE' ) );
#7985=VERTEX_POINT ( 'NONE', #10489 ) ;
#7988=EDGE_CURVE ( 'NONE', #8980, #8709, #7204, .T. ) ;
#7989=DIRECTION ( 'NONE',  ( 1.000000000000000000, -0.000000000000000000, -0.000000000000000000 ) ) ;
#7994=( LENGTH_UNIT ( ) NAMED_UNIT ( * ) SI_UNIT ( .MILLI., .METRE. ) );
#7995=CYLINDRICAL_SURFACE ( 'NONE', #8565, 3.500000000000003109 ) ;
#7996=ADVANCED_FACE ( 'NONE', ( #3436 ), #8600, .F. ) ;
#8003=AXIS2_PLACEMENT_3D ( 'NONE', #1767, #5756, #12505 ) ;
#8007=UNCERTAINTY_MEASURE_WITH_UNIT (LENGTH_MEASURE( 1.000000000000000082E-05 ), #7207, 'distance_accuracy_value', 'NONE');
#8026=LINE ( 'NONE', #11943, #4664 ) ;
#8038=ORIENTED_EDGE ( 'NONE', *, *, #9088, .F. ) ;
#8042=ORIENTED_EDGE ( 'NONE', *, *, #12633, .T. ) ;
#8043=DIRECTION ( 'NONE',  ( -1.000000000000000000, 0.000000000000000000, 0.000000000000000000 ) ) ;
#8044=CARTESIAN_POINT ( 'NONE',  ( 21.49999999999998579, 90.00000000000000000, -10.00000000000000178 ) ) ;
#8063=FACE_BOUND ( 'NONE', #4231, .T. ) ;
#8075=EDGE_CURVE ( 'NONE', #5822, #4697, #3568, .T. ) ;
#8085=DIRECTION ( 'NONE',  ( -0.000000000000000000, -0.000000000000000000, -1.000000000000000000 ) ) ;
#8095=ADVANCED_BREP_SHAPE_REPRESENTATION ( '', ( #11745, #5704 ), #898 ) ;
#8096=CARTESIAN_POINT ( 'NONE',  ( 35.00000000000000000, 90.00000000000000000, 4.000000000000000000 ) ) ;
#8124=EDGE_CURVE ( 'NONE', #7014, #8561, #4491, .T. ) ;
#8138=CARTESIAN_POINT ( 'NONE',  ( 21.49999999999998579, 90.00000000000000000, -10.00000000000000000 ) ) ;
#8139=CARTESIAN_POINT ( 'NONE',  ( 38.50000000000000711, 90.00000000000000000, 6.000000000000000000 ) ) ;
#8144=CARTESIAN_POINT ( 'NONE',  ( 35.75000000000000711, 93.41869858279433458, 6.000000000000000000 ) ) ;
#8145=DIRECTION ( 'NONE',  ( -1.000000000000000000, 0.000000000000000000, 0.000000000000000000 ) ) ;
#8147=CARTESIAN_POINT ( 'NONE',  ( 35.00000000000000000, 90.00000000000000000, -8.000000000000000000 ) ) ;
#8151=LINE ( 'NONE', #12863, #11284 ) ;
#8154=VECTOR ( 'NONE', #12497, 1000.000000000000000 ) ;
#8160=EDGE_CURVE ( 'NONE', #11257, #8414, #11799, .T. ) ;
#8163=AXIS2_PLACEMENT_3D ( 'NONE', #5981, #5199, #2068 ) ;
#8165=LINE ( 'NONE', #8421, #3469 ) ;
#8175=ORIENTED_EDGE ( 'NONE', *, *, #12241, .F. ) ;
#8183=DIRECTION ( 'NONE',  ( -1.000000000000000000, 0.000000000000000000, 0.000000000000000000 ) ) ;
#8188=LINE ( 'NONE', #12175, #5479 ) ;
#8190=MECHANICAL_DESIGN_GEOMETRIC_PRESENTATION_REPRESENTATION('',(#6706),#7981);
#8201=CIRCLE ( 'NONE', #8621, 4.000000000000003553 ) ;
#8207=CYLINDRICAL_SURFACE ( 'NONE', #6653, 3.500000000000003109 ) ;
#8211=LINE ( 'NONE', #2265, #4402 ) ;
#8214=CARTESIAN_POINT ( 'NONE',  ( 35.00000000000000000, 90.00000000000000000, 6.000000000000000000 ) ) ;
#8223=CARTESIAN_POINT ( 'NONE',  ( 36.58116973490655255, 87.04662866042625069, -3.799999999999999822 ) ) ;
#8230=LINE ( 'NONE', #297, #6391 ) ;
#8236=CARTESIAN_POINT ( 'NONE',  ( 52.49999999999996447, 94.00000000000000000, -8.000000000000000000 ) ) ;
#8256=PRESENTATION_STYLE_ASSIGNMENT (( #5430 ) ) ;
#8257=DIRECTION ( 'NONE',  ( -1.000000000000000000, 0.000000000000000000, 0.000000000000000000 ) ) ;
#8266=FACE_OUTER_BOUND ( 'NONE', #4247, .T. ) ;
#8286=EDGE_CURVE ( 'NONE', #5406, #9676, #3488, .T. ) ;
#8299=DIRECTION ( 'NONE',  ( 0.000000000000000000, 0.000000000000000000, 1.000000000000000000 ) ) ;
#8316=EDGE_LOOP ( 'NONE', ( #12352, #5950, #12954, #3254, #12378 ) ) ;
#8317=CARTESIAN_POINT ( 'NONE',  ( 34.25000000000000000, 93.41869858279433458, 6.000000000000000000 ) ) ;
#8328=VECTOR ( 'NONE', #4654, 1000.000000000000000 ) ;
#8329=ORIENTED_EDGE ( 'NONE', *, *, #1489, .F. ) ;
#8341=DIRECTION ( 'NONE',  ( 5.624500927088228034E-17, -1.370729058197317775E-18, -1.000000000000000000 ) ) ;
#8343=AXIS2_PLACEMENT_3D ( 'NONE', #9830, #9958, #796 ) ;
#8363=CIRCLE ( 'NONE', #400, 3.500000000000003109 ) ;
#8367=EDGE_LOOP ( 'NONE', ( #6293, #5211, #88, #1372 ) ) ;
#8375=CARTESIAN_POINT ( 'NONE',  ( 34.25000000000000000, 93.41869858279433458, -3.799999999999999378 ) ) ;
#8382=DIRECTION ( 'NONE',  ( 0.000000000000000000, 0.000000000000000000, -1.000000000000000000 ) ) ;
#8393=EDGE_CURVE ( 'NONE', #1694, #29, #843, .T. ) ;
#8404=DIRECTION ( 'NONE',  ( 0.000000000000000000, -0.000000000000000000, 1.000000000000000000 ) ) ;
#8408=LINE ( 'NONE', #5651, #11183 ) ;
#8409=DIRECTION ( 'NONE',  ( 0.000000000000000000, 0.000000000000000000, 1.000000000000000000 ) ) ;
#8414=VERTEX_POINT ( 'NONE', #4848 ) ;
#8421=CARTESIAN_POINT ( 'NONE',  ( 38.50000000000000711, 90.00000000000000000, 6.000000000000000000 ) ) ;
#8422=DIRECTION ( 'NONE',  ( -1.000000000000000000, 0.000000000000000000, 0.000000000000000000 ) ) ;
#8428=ORIENTED_EDGE ( 'NONE', *, *, #11483, .T. ) ;
#8448=CARTESIAN_POINT ( 'NONE',  ( 35.75000000000000711, 92.49999999999998579, 4.000000000000000000 ) ) ;
#8449=VECTOR ( 'NONE', #12200, 1000.000000000000000 ) ;
#8461=VECTOR ( 'NONE', #6560, 1000.000000000000000 ) ;
#8471=DIRECTION ( 'NONE',  ( -0.9549484348006340717, -0.2967717757331703732, 0.000000000000000000 ) ) ;
#8472=DIRECTION ( 'NONE',  ( -0.3262398754384822630, 0.9452870165584014162, 0.000000000000000000 ) ) ;
#8473=FACE_OUTER_BOUND ( 'NONE', #11176, .T. ) ;
#8474=EDGE_CURVE ( 'NONE', #5822, #294, #5536, .T. ) ;
#8481=DIRECTION ( 'NONE',  ( 1.000000000000000000, 0.000000000000000000, -0.000000000000000000 ) ) ;
#8495=DIRECTION ( 'NONE',  ( -1.000000000000000000, 0.000000000000000000, 0.000000000000000000 ) ) ;
#8498=ORIENTED_EDGE ( 'NONE', *, *, #10591, .F. ) ;
#8501=CARTESIAN_POINT ( 'NONE',  ( 35.75000000000000711, 93.41869858279433458, 6.000000000000000000 ) ) ;
#8511=VERTEX_POINT ( 'NONE', #10004 ) ;
#8539=CARTESIAN_POINT ( 'NONE',  ( 52.49999999999996447, 86.00000000000000000, -10.00000000000000000 ) ) ;
#8547=DIRECTION ( 'NONE',  ( 0.4719909656437444867, -0.8816033849473842166, 0.000000000000000000 ) ) ;
#8551=CARTESIAN_POINT ( 'NONE',  ( 35.00000000000000000, 90.00000000000000000, -10.00000000000000000 ) ) ;
#8552=DIRECTION ( 'NONE',  ( 0.000000000000000000, -0.000000000000000000, -1.000000000000000000 ) ) ;
#8556=DIRECTION ( 'NONE',  ( -1.000000000000000000, 0.000000000000000000, 0.000000000000000000 ) ) ;
#8561=VERTEX_POINT ( 'NONE', #10129 ) ;
#8562=CIRCLE ( 'NONE', #4802, 1.599999999999990319 ) ;
#8565=AXIS2_PLACEMENT_3D ( 'NONE', #1183, #4269, #8257 ) ;
#8571=VERTEX_POINT ( 'NONE', #11502 ) ;
#8582=PLANE ( 'NONE',  #358 ) ;
#8600=PLANE ( 'NONE',  #12423 ) ;
#8607=DIRECTION ( 'NONE',  ( 0.9347165045408831752, 0.3553942263724512163, 0.000000000000000000 ) ) ;
#8609=DIRECTION ( 'NONE',  ( -5.624500927088228034E-17, 1.370729058197317775E-18, 1.000000000000000000 ) ) ;
#8619=CARTESIAN_POINT ( 'NONE',  ( 48.49999999999995737, 90.00000000000000000, -10.00000000000000178 ) ) ;
#8621=AXIS2_PLACEMENT_3D ( 'NONE', #9097, #981, #12835 ) ;
#8623=ORIENTED_EDGE ( 'NONE', *, *, #12906, .T. ) ;
#8624=DIRECTION ( 'NONE',  ( -1.000000000000000000, 0.000000000000000000, 0.000000000000000000 ) ) ;
#8629=VECTOR ( 'NONE', #8043, 1000.000000000000000 ) ;
#8631=VERTEX_POINT ( 'NONE', #8375 ) ;
#8639=EDGE_CURVE ( 'NONE', #9191, #4447, #6331, .T. ) ;
#8644=AXIS2_PLACEMENT_3D ( 'NONE', #9894, #67, #11128 ) ;
#8646=EDGE_LOOP ( 'NONE', ( #10614, #9395, #2289, #9111 ) ) ;
#8662=CARTESIAN_POINT ( 'NONE',  ( 45.00000000000000711, 90.00000000000000000, -18.00000000000000355 ) ) ;
#8684=EDGE_CURVE ( 'NONE', #12608, #4194, #9410, .T. ) ;
#8698=EDGE_LOOP ( 'NONE', ( #2624, #10635, #8038, #4375 ) ) ;
#8702=ORIENTED_EDGE ( 'NONE', *, *, #8982, .T. ) ;
#8706=EDGE_CURVE ( 'NONE', #7837, #12083, #9093, .T. ) ;
#8709=VERTEX_POINT ( 'NONE', #7452 ) ;
#8710=PLANE ( 'NONE',  #3974 ) ;
#8714=DIRECTION ( 'NONE',  ( -5.624500927088228034E-17, 1.370729058197317775E-18, 1.000000000000000000 ) ) ;
#8720=EDGE_CURVE ( 'NONE', #2378, #5783, #8880, .T. ) ;
#8731=CARTESIAN_POINT ( 'NONE',  ( 31.80092274341787828, 89.00581455129388075, 4.800000000000000711 ) ) ;
#8740=VECTOR ( 'NONE', #10259, 1000.000000000000000 ) ;
#8748=CIRCLE ( 'NONE', #6446, 10.00000000000000178 ) ;
#8756=ORIENTED_EDGE ( 'NONE', *, *, #5082, .F. ) ;
#8760=DIRECTION ( 'NONE',  ( 1.000000000000000000, 0.000000000000000000, 0.000000000000000000 ) ) ;
#8762=AXIS2_PLACEMENT_3D ( 'NONE', #5649, #3633, #8471 ) ;
#8769=ADVANCED_FACE ( 'NONE', ( #8815 ), #10594, .T. ) ;
#8774=CARTESIAN_POINT ( 'NONE',  ( 21.49999999999998579, 90.00000000000000000, -8.000000000000000000 ) ) ;
#8778=AXIS2_PLACEMENT_3D ( 'NONE', #11358, #2410, #8556 ) ;
#8780=DIRECTION ( 'NONE',  ( 0.000000000000000000, 0.000000000000000000, -1.000000000000000000 ) ) ;
#8786=DIRECTION ( 'NONE',  ( 1.000000000000000000, 0.000000000000000000, 0.000000000000000000 ) ) ;
#8796=VECTOR ( 'NONE', #1124, 1000.000000000000000 ) ;
#8815=FACE_OUTER_BOUND ( 'NONE', #4051, .T. ) ;
#8850=VECTOR ( 'NONE', #3195, 1000.000000000000000 ) ;
#8856=EDGE_CURVE ( 'NONE', #6452, #2378, #12876, .T. ) ;
#8879=EDGE_CURVE ( 'NONE', #3957, #2378, #12760, .T. ) ;
#8880=CIRCLE ( 'NONE', #12856, 3.500000000000003109 ) ;
#8882=ORIENTED_EDGE ( 'NONE', *, *, #11025, .T. ) ;
#8894=EDGE_LOOP ( 'NONE', ( #2865, #5696 ) ) ;
#8898=CARTESIAN_POINT ( 'NONE',  ( 35.00000000000000000, 90.00000000000000000, 6.000000000000000000 ) ) ;
#8908=VERTEX_POINT ( 'NONE', #6302 ) ;
#8926=ADVANCED_FACE ( 'NONE', ( #6106 ), #10295, .T. ) ;
#8934=ORIENTED_EDGE ( 'NONE', *, *, #9832, .T. ) ;
#8941=ORIENTED_EDGE ( 'NONE', *, *, #3607, .T. ) ;
#8942=DIRECTION ( 'NONE',  ( 0.000000000000000000, 0.000000000000000000, -1.000000000000000000 ) ) ;
#8951=EDGE_CURVE ( 'NONE', #8561, #1735, #2074, .T. ) ;
#8955=EDGE_LOOP ( 'NONE', ( #3749, #1126, #5947, #706, #6527, #11704 ) ) ;
#8969=FACE_OUTER_BOUND ( 'NONE', #6668, .T. ) ;
#8975=ORIENTED_EDGE ( 'NONE', *, *, #4903, .T. ) ;
#8980=VERTEX_POINT ( 'NONE', #5195 ) ;
#8982=EDGE_CURVE ( 'NONE', #5937, #9364, #5323, .T. ) ;
#8986=EDGE_CURVE ( 'NONE', #216, #4697, #4992, .T. ) ;
#8993=ORIENTED_EDGE ( 'NONE', *, *, #3565, .T. ) ;
#8997=CARTESIAN_POINT ( 'NONE',  ( 0.000000000000000000, 0.000000000000000000, 0.000000000000000000 ) ) ;
#9006=CARTESIAN_POINT ( 'NONE',  ( 35.75000000000000711, 92.49999999999998579, -8.000000000000000000 ) ) ;
#9007=ORIENTED_EDGE ( 'NONE', *, *, #9115, .F. ) ;
#9013=CARTESIAN_POINT ( 'NONE',  ( 31.80092274341787828, 89.00581455129388075, 4.000000000000000000 ) ) ;
#9019=VECTOR ( 'NONE', #121, 1000.000000000000000 ) ;
#9024=EDGE_CURVE ( 'NONE', #6329, #3747, #8211, .T. ) ;
#9030=CIRCLE ( 'NONE', #2986, 3.350000000000003642 ) ;
#9034=EDGE_LOOP ( 'NONE', ( #11231, #11174, #9458, #5291 ) ) ;
#9042=ORIENTED_EDGE ( 'NONE', *, *, #12906, .F. ) ;
#9054=AXIS2_PLACEMENT_3D ( 'NONE', #7489, #10432, #7358 ) ;
#9055=DIRECTION ( 'NONE',  ( 0.000000000000000000, -1.000000000000000000, 0.000000000000000000 ) ) ;
#9057=EDGE_CURVE ( 'NONE', #4963, #12297, #1661, .T. ) ;
#9070=DIRECTION ( 'NONE',  ( 0.000000000000000000, -1.000000000000000000, -0.000000000000000000 ) ) ;
#9083=ORIENTED_EDGE ( 'NONE', *, *, #8286, .F. ) ;
#9088=EDGE_CURVE ( 'NONE', #3524, #7014, #10685, .T. ) ;
#9093=CIRCLE ( 'NONE', #1141, 3.349999999999995204 ) ;
#9097=CARTESIAN_POINT ( 'NONE',  ( 48.49999999999995737, 90.00000000000000000, -8.000000000000000000 ) ) ;
#9101=EDGE_LOOP ( 'NONE', ( #12050, #6352, #12313, #1936, #151, #7716, #650, #11784 ) ) ;
#9111=ORIENTED_EDGE ( 'NONE', *, *, #5699, .F. ) ;
#9115=EDGE_CURVE ( 'NONE', #655, #11127, #2581, .T. ) ;
#9117=ADVANCED_FACE ( 'NONE', ( #10428 ), #9512, .F. ) ;
#9119=DIRECTION ( 'NONE',  ( 0.000000000000000000, 0.000000000000000000, 1.000000000000000000 ) ) ;
#9123=FACE_OUTER_BOUND ( 'NONE', #4439, .T. ) ;
#9125=VERTEX_POINT ( 'NONE', #10490 ) ;
#9133=ORIENTED_EDGE ( 'NONE', *, *, #12555, .T. ) ;
#9151=SHAPE_DEFINITION_REPRESENTATION ( #12421, #5582 ) ;
#9157=DIRECTION ( 'NONE',  ( -0.000000000000000000, -0.000000000000000000, -1.000000000000000000 ) ) ;
#9159=CARTESIAN_POINT ( 'NONE',  ( 31.86869970978804290, 88.80942934165229019, 4.800000000000000711 ) ) ;
#9164=AXIS2_PLACEMENT_3D ( 'NONE', #3352, #6405, #5166 ) ;
#9169=ORIENTED_EDGE ( 'NONE', *, *, #12451, .T. ) ;
#9177=AXIS2_PLACEMENT_3D ( 'NONE', #12115, #1311, #5547 ) ;
#9179=PLANE ( 'NONE',  #10406 ) ;
#9185=CARTESIAN_POINT ( 'NONE',  ( 31.65768047819777919, 88.96129878493390208, 4.800000000000000711 ) ) ;
#9191=VERTEX_POINT ( 'NONE', #3953 ) ;
#9197=CARTESIAN_POINT ( 'NONE',  ( 31.86869970978804290, 88.80942934165229019, 4.800000000000000711 ) ) ;
#9202=DIRECTION ( 'NONE',  ( -0.3262398754384820410, 0.9452870165584015272, 0.000000000000000000 ) ) ;
#9205=DIRECTION ( 'NONE',  ( 0.4719909656437444867, -0.8816033849473842166, 0.000000000000000000 ) ) ;
#9220=ADVANCED_FACE ( 'NONE', ( #10022 ), #4987, .F. ) ;
#9228=PLANE ( 'NONE',  #581 ) ;
#9238=EDGE_CURVE ( 'NONE', #4244, #7837, #2968, .T. ) ;
#9267=ORIENTED_EDGE ( 'NONE', *, *, #5434, .F. ) ;
#9273=DIRECTION ( 'NONE',  ( 1.000000000000000000, -0.000000000000000000, -0.000000000000000000 ) ) ;
#9281=EDGE_CURVE ( 'NONE', #370, #12297, #1235, .T. ) ;
#9300=ORIENTED_EDGE ( 'NONE', *, *, #9802, .F. ) ;
#9313=CARTESIAN_POINT ( 'NONE',  ( 44.16515138991168499, 94.00000000000000000, -10.00000000000000000 ) ) ;
#9319=CARTESIAN_POINT ( 'NONE',  ( 35.00000000000000000, 90.00000000000000000, 4.800000000000000711 ) ) ;
#9322=CIRCLE ( 'NONE', #6812, 1.599999999999990319 ) ;
#9361=DIRECTION ( 'NONE',  ( 1.000000000000000000, 0.000000000000000000, 0.000000000000000000 ) ) ;
#9364=VERTEX_POINT ( 'NONE', #11200 ) ;
#9375=CARTESIAN_POINT ( 'NONE',  ( 35.75000000000000711, 93.41869858279433458, -3.000000000000000000 ) ) ;
#9383=AXIS2_PLACEMENT_3D ( 'NONE', #3096, #7075, #2110 ) ;
#9395=ORIENTED_EDGE ( 'NONE', *, *, #7547, .T. ) ;
#9396=CARTESIAN_POINT ( 'NONE',  ( 48.49999999999995737, 90.00000000000000000, -8.000000000000000000 ) ) ;
#9401=ORIENTED_EDGE ( 'NONE', *, *, #3904, .F. ) ;
#9410=LINE ( 'NONE', #3536, #1789 ) ;
#9416=CARTESIAN_POINT ( 'NONE',  ( 35.00000000000000000, 90.00000000000000000, -8.000000000000000000 ) ) ;
#9423=DIRECTION ( 'NONE',  ( -1.000000000000000000, 0.000000000000000000, -0.000000000000000000 ) ) ;
#9445=LINE ( 'NONE', #8662, #3664 ) ;
#9451=DIRECTION ( 'NONE',  ( 1.000000000000000000, 0.000000000000000000, 0.000000000000000000 ) ) ;
#9458=ORIENTED_EDGE ( 'NONE', *, *, #9473, .F. ) ;
#9473=EDGE_CURVE ( 'NONE', #11514, #8561, #12052, .T. ) ;
#9508=CIRCLE ( 'NONE', #7212, 4.000000000000003553 ) ;
#9512=PLANE ( 'NONE',  #8762 ) ;
#9533=CYLINDRICAL_SURFACE ( 'NONE', #8778, 1.599999999999990319 ) ;
#9540=VECTOR ( 'NONE', #12322, 1000.000000000000000 ) ;
#9541=DIRECTION ( 'NONE',  ( 0.000000000000000000, 0.000000000000000000, -1.000000000000000000 ) ) ;
#9548=ORIENTED_EDGE ( 'NONE', *, *, #11025, .F. ) ;
#9556=ORIENTED_EDGE ( 'NONE', *, *, #7447, .T. ) ;
#9571=CARTESIAN_POINT ( 'NONE',  ( 33.90709641728108892, 93.16671150547063007, 4.800000000000000711 ) ) ;
#9599=ORIENTED_EDGE ( 'NONE', *, *, #4872, .T. ) ;
#9606=LINE ( 'NONE', #11755, #5625 ) ;
#9618=( NAMED_UNIT ( * ) SI_UNIT ( $, .STERADIAN. ) SOLID_ANGLE_UNIT ( ) );
#9627=VERTEX_POINT ( 'NONE', #7535 ) ;
#9638=CARTESIAN_POINT ( 'NONE',  ( 35.00000000000000000, 90.00000000000000000, -3.000000000000000000 ) ) ;
#9642=FACE_OUTER_BOUND ( 'NONE', #8646, .T. ) ;
#9646=FACE_OUTER_BOUND ( 'NONE', #2037, .T. ) ;
#9648=DIRECTION ( 'NONE',  ( 1.000000000000000000, 0.000000000000000000, 0.000000000000000000 ) ) ;
#9660=VERTEX_POINT ( 'NONE', #1712 ) ;
#9662=CARTESIAN_POINT ( 'NONE',  ( 52.49999999999996447, 90.00000000000000000, -8.000000000000000000 ) ) ;
#9664=ADVANCED_FACE ( 'NONE', ( #4972 ), #10918, .T. ) ;
#9670=ORIENTED_EDGE ( 'NONE', *, *, #9473, .T. ) ;
#9676=VERTEX_POINT ( 'NONE', #11779 ) ;
#9677=( LENGTH_UNIT ( ) NAMED_UNIT ( * ) SI_UNIT ( .MILLI., .METRE. ) );
#9680=EDGE_CURVE ( 'NONE', #8908, #10536, #8562, .T. ) ;
#9682=DIRECTION ( 'NONE',  ( -0.000000000000000000, -0.000000000000000000, -1.000000000000000000 ) ) ;
#9693=CARTESIAN_POINT ( 'NONE',  ( 34.25000000000000000, 93.26496554346289258, -3.000000000000000000 ) ) ;
#9709=DIRECTION ( 'NONE',  ( 0.9347165045408831752, 0.3553942263724512163, 0.000000000000000000 ) ) ;
#9712=EDGE_CURVE ( 'NONE', #3747, #9191, #393, .T. ) ;
#9718=PLANE ( 'NONE',  #4090 ) ;
#9723=ORIENTED_EDGE ( 'NONE', *, *, #4458, .T. ) ;
#9725=EDGE_LOOP ( 'NONE', ( #9548, #11381, #4387, #10782, #10581 ) ) ;
#9735=CARTESIAN_POINT ( 'NONE',  ( 31.50000000000000000, 90.00000000000000000, 6.000000000000000000 ) ) ;
#9736=ORIENTED_EDGE ( 'NONE', *, *, #705, .F. ) ;
#9745=ORIENTED_EDGE ( 'NONE', *, *, #9712, .T. ) ;
#9755=ADVANCED_FACE ( 'NONE', ( #719 ), #8710, .T. ) ;
#9766=DIRECTION ( 'NONE',  ( 1.000000000000000000, 0.000000000000000000, 0.000000000000000000 ) ) ;
#9774=ORIENTED_EDGE ( 'NONE', *, *, #3660, .T. ) ;
#9776=CARTESIAN_POINT ( 'NONE',  ( 31.86869970978804290, 88.80942934165229019, 4.800000000000000711 ) ) ;
#9796=FACE_OUTER_BOUND ( 'NONE', #2855, .T. ) ;
#9801=DIRECTION ( 'NONE',  ( -1.000000000000000000, -2.081668171172168513E-14, 0.000000000000000000 ) ) ;
#9802=EDGE_CURVE ( 'NONE', #7980, #3747, #507, .T. ) ;
#9811=LINE ( 'NONE', #5878, #8328 ) ;
#9818=ORIENTED_EDGE ( 'NONE', *, *, #9680, .T. ) ;
#9830=CARTESIAN_POINT ( 'NONE',  ( 35.00000000000000000, 90.00000000000000000, 4.000000000000000000 ) ) ;
#9832=EDGE_CURVE ( 'NONE', #9660, #4244, #11701, .T. ) ;
#9833=DIRECTION ( 'NONE',  ( 0.4719909656437442647, -0.8816033849473842166, 2.775557561595757269E-17 ) ) ;
#9846=CARTESIAN_POINT ( 'NONE',  ( 35.00000000000000000, 90.00000000000000000, 6.000000000000000000 ) ) ;
#9872=ADVANCED_FACE ( 'NONE', ( #10904 ), #5746, .T. ) ;
#9876=DIRECTION ( 'NONE',  ( 1.000000000000000000, 0.000000000000000000, 0.000000000000000000 ) ) ;
#9885=VECTOR ( 'NONE', #1777, 1000.000000000000000 ) ;
#9889=CARTESIAN_POINT ( 'NONE',  ( 35.00000000000000000, 90.00000000000000000, -10.00000000000000000 ) ) ;
#9892=VERTEX_POINT ( 'NONE', #12689 ) ;
#9894=CARTESIAN_POINT ( 'NONE',  ( 52.49999999999996447, 86.00000000000000000, -10.00000000000000000 ) ) ;
#9917=CARTESIAN_POINT ( 'NONE',  ( 38.50000000000000711, 90.00000000000000000, -3.000000000000000888 ) ) ;
#9934=EDGE_CURVE ( 'NONE', #9892, #11514, #1883, .T. ) ;
#9936=DIRECTION ( 'NONE',  ( -0.9549484348006339607, -0.2967717757331703732, 0.000000000000000000 ) ) ;
#9948=ORIENTED_EDGE ( 'NONE', *, *, #8474, .T. ) ;
#9958=DIRECTION ( 'NONE',  ( 0.000000000000000000, 0.000000000000000000, -1.000000000000000000 ) ) ;
#9970=AXIS2_PLACEMENT_3D ( 'NONE', #5785, #12727, #6958 ) ;
#9978=VECTOR ( 'NONE', #187, 1000.000000000000000 ) ;
#9980=ORIENTED_EDGE ( 'NONE', *, *, #10170, .F. ) ;
#9988=AXIS2_PLACEMENT_3D ( 'NONE', #7721, #11900, #777 ) ;
#10004=CARTESIAN_POINT ( 'NONE',  ( 36.58116973490655255, 87.04662866042625069, -3.799999999999999822 ) ) ;
#10022=FACE_OUTER_BOUND ( 'NONE', #2152, .T. ) ;
#10024=ORIENTED_EDGE ( 'NONE', *, *, #48, .T. ) ;
#10059=CARTESIAN_POINT ( 'NONE',  ( 36.58116973490655255, 87.04662866042625069, -3.000000000000000000 ) ) ;
#10064=EDGE_LOOP ( 'NONE', ( #181, #3147, #3008, #12027 ) ) ;
#10067=ORIENTED_EDGE ( 'NONE', *, *, #4050, .T. ) ;
#10071=EDGE_CURVE ( 'NONE', #2177, #4130, #11094, .T. ) ;
#10087=AXIS2_PLACEMENT_3D ( 'NONE', #885, #823, #4889 ) ;
#10090=ORIENTED_EDGE ( 'NONE', *, *, #6103, .F. ) ;
#10093=EDGE_CURVE ( 'NONE', #6329, #5120, #6121, .T. ) ;
#10098=CARTESIAN_POINT ( 'NONE',  ( 35.00000000000000000, 90.00000000000000000, -8.000000000000000000 ) ) ;
#10099=LINE ( 'NONE', #12135, #8449 ) ;
#10102=EDGE_CURVE ( 'NONE', #10917, #2666, #12548, .T. ) ;
#10103=FACE_OUTER_BOUND ( 'NONE', #1166, .T. ) ;
#10115=DIRECTION ( 'NONE',  ( -0.000000000000000000, -0.000000000000000000, -1.000000000000000000 ) ) ;
#10116=DIRECTION ( 'NONE',  ( -0.000000000000000000, -0.000000000000000000, 1.000000000000000000 ) ) ;
#10124=LINE ( 'NONE', #11172, #12511 ) ;
#10129=CARTESIAN_POINT ( 'NONE',  ( 17.49999999999998579, 90.00000000000002842, -10.00000000000000000 ) ) ;
#10136=CARTESIAN_POINT ( 'NONE',  ( 52.49999999999996447, 86.00000000000000000, -10.00000000000000000 ) ) ;
#10146=PLANE ( 'NONE',  #1658 ) ;
#10150=AXIS2_PLACEMENT_3D ( 'NONE', #7374, #3272, #11362 ) ;
#10162=CARTESIAN_POINT ( 'NONE',  ( 44.16515138991168499, 94.00000000000000000, -8.000000000000000000 ) ) ;
#10167=CARTESIAN_POINT ( 'NONE',  ( 35.00000000000000000, 90.00000000000000000, 4.800000000000000711 ) ) ;
#10170=EDGE_CURVE ( 'NONE', #11127, #1353, #8363, .T. ) ;
#10180=APPLICATION_CONTEXT ( 'automotive_design' ) ;
#10185=CARTESIAN_POINT ( 'NONE',  ( 44.16515138991168499, 94.00000000000000000, -18.00000000000000355 ) ) ;
#10197=ADVANCED_FACE ( 'NONE', ( #2344 ), #9533, .F. ) ;
#10203=ORIENTED_EDGE ( 'NONE', *, *, #10639, .F. ) ;
#10205=PLANE ( 'NONE',  #3961 ) ;
#10215=AXIS2_PLACEMENT_3D ( 'NONE', #4410, #463, #3501 ) ;
#10220=EDGE_LOOP ( 'NONE', ( #12702, #7037, #10336, #9007 ) ) ;
#10222=DIRECTION ( 'NONE',  ( -5.624500927088228034E-17, 1.370729058197317968E-18, 1.000000000000000000 ) ) ;
#10236=DIRECTION ( 'NONE',  ( 0.000000000000000000, 0.000000000000000000, -1.000000000000000000 ) ) ;
#10242=VECTOR ( 'NONE', #10236, 1000.000000000000000 ) ;
#10250=DIRECTION ( 'NONE',  ( -1.000000000000000000, 0.000000000000000000, 0.000000000000000000 ) ) ;
#10258=AXIS2_PLACEMENT_3D ( 'NONE', #8138, #2911, #12849 ) ;
#10259=DIRECTION ( 'NONE',  ( 0.000000000000000000, 0.000000000000000000, 1.000000000000000000 ) ) ;
#10263=DIRECTION ( 'NONE',  ( 1.000000000000000000, 0.000000000000000000, 0.000000000000000000 ) ) ;
#10295=CYLINDRICAL_SURFACE ( 'NONE', #7085, 4.000000000000003553 ) ;
#10296=LINE ( 'NONE', #4096, #3019 ) ;
#10307=LINE ( 'NONE', #2339, #6358 ) ;
#10319=EDGE_LOOP ( 'NONE', ( #9267, #7773, #10394, #8941 ) ) ;
#10321=ORIENTED_EDGE ( 'NONE', *, *, #5434, .T. ) ;
#10336=ORIENTED_EDGE ( 'NONE', *, *, #12589, .T. ) ;
#10366=LINE ( 'NONE', #11606, #11151 ) ;
#10370=LINE ( 'NONE', #5453, #2449 ) ;
#10371=ORIENTED_EDGE ( 'NONE', *, *, #7988, .F. ) ;
#10372=CARTESIAN_POINT ( 'NONE',  ( 35.00000000000000000, 90.00000000000000000, -3.799999999999999822 ) ) ;
#10377=DIRECTION ( 'NONE',  ( -1.000000000000000000, 0.000000000000000000, 0.000000000000000000 ) ) ;
#10381=CARTESIAN_POINT ( 'NONE',  ( 48.49999999999995737, 90.00000000000000000, -8.000000000000000000 ) ) ;
#10394=ORIENTED_EDGE ( 'NONE', *, *, #5749, .T. ) ;
#10406=AXIS2_PLACEMENT_3D ( 'NONE', #7221, #5122, #11209 ) ;
#10411=ORIENTED_EDGE ( 'NONE', *, *, #4903, .F. ) ;
#10420=CARTESIAN_POINT ( 'NONE',  ( 31.96709571323326671, 88.25314809233525182, -3.000000000000000888 ) ) ;
#10423=CARTESIAN_POINT ( 'NONE',  ( 31.50000000000000000, 90.00000000000000000, -3.799999999999999378 ) ) ;
#10428=FACE_OUTER_BOUND ( 'NONE', #10220, .T. ) ;
#10432=DIRECTION ( 'NONE',  ( -0.000000000000000000, 0.000000000000000000, -1.000000000000000000 ) ) ;
#10439=AXIS2_PLACEMENT_3D ( 'NONE', #10996, #2777, #5841 ) ;
#10445=CARTESIAN_POINT ( 'NONE',  ( 35.00000000000000000, 90.00000000000000000, 4.800000000000000711 ) ) ;
#10447=ORIENTED_EDGE ( 'NONE', *, *, #8393, .F. ) ;
#10453=ORIENTED_EDGE ( 'NONE', *, *, #3925, .T. ) ;
#10454=ADVANCED_FACE ( 'NONE', ( #9123 ), #7955, .T. ) ;
#10460=DIRECTION ( 'NONE',  ( 1.000000000000000000, 0.000000000000000000, 0.000000000000000000 ) ) ;
#10465=ORIENTED_EDGE ( 'NONE', *, *, #5511, .T. ) ;
#10478=ADVANCED_FACE ( 'NONE', ( #10103 ), #11937, .T. ) ;
#10485=VECTOR ( 'NONE', #9451, 1000.000000000000000 ) ;
#10489=CARTESIAN_POINT ( 'NONE',  ( 25.83484861008832567, 94.00000000000000000, -8.000000000000000000 ) ) ;
#10490=CARTESIAN_POINT ( 'NONE',  ( 35.75000000000000711, 93.41869858279433458, 4.000000000000000000 ) ) ;
#10498=FACE_OUTER_BOUND ( 'NONE', #3677, .T. ) ;
#10504=CARTESIAN_POINT ( 'NONE',  ( 31.99902028769960438, 88.51116798584881451, -3.800000000000000266 ) ) ;
#10507=ADVANCED_FACE ( 'NONE', ( #2133 ), #6109, .F. ) ;
#10530=EDGE_CURVE ( 'NONE', #4697, #7837, #1136, .T. ) ;
#10536=VERTEX_POINT ( 'NONE', #13 ) ;
#10556=EDGE_CURVE ( 'NONE', #6404, #9125, #8151, .T. ) ;
#10568=CARTESIAN_POINT ( 'NONE',  ( 34.25000000000000000, 93.41869858279433458, -8.000000000000000000 ) ) ;
#10571=FACE_OUTER_BOUND ( 'NONE', #8955, .T. ) ;
#10575=AXIS2_PLACEMENT_3D ( 'NONE', #3507, #10936, #9833 ) ;
#10581=ORIENTED_EDGE ( 'NONE', *, *, #2406, .F. ) ;
#10586=EDGE_LOOP ( 'NONE', ( #12349, #4560, #11734, #4299, #12479, #12612 ) ) ;
#10591=EDGE_CURVE ( 'NONE', #1353, #11880, #6046, .T. ) ;
#10592=LINE ( 'NONE', #636, #5089 ) ;
#10594=CYLINDRICAL_SURFACE ( 'NONE', #5405, 3.500000000000003109 ) ;
#10595=ORIENTED_EDGE ( 'NONE', *, *, #12775, .T. ) ;
#10610=ORIENTED_EDGE ( 'NONE', *, *, #2406, .T. ) ;
#10614=ORIENTED_EDGE ( 'NONE', *, *, #9680, .F. ) ;
#10631=CARTESIAN_POINT ( 'NONE',  ( 0.000000000000000000, 0.000000000000000000, -10.00000000000000000 ) ) ;
#10635=ORIENTED_EDGE ( 'NONE', *, *, #11013, .T. ) ;
#10639=EDGE_CURVE ( 'NONE', #7985, #485, #6308, .T. ) ;
#10645=VERTEX_POINT ( 'NONE', #6245 ) ;
#10647=LINE ( 'NONE', #1624, #5818 ) ;
#10655=CARTESIAN_POINT ( 'NONE',  ( 21.49999999999998579, 90.00000000000000000, -8.000000000000000000 ) ) ;
#10663=VECTOR ( 'NONE', #11878, 1000.000000000000000 ) ;
#10685=LINE ( 'NONE', #8539, #12096 ) ;
#10687=DIRECTION ( 'NONE',  ( -1.000000000000000000, 0.000000000000000000, 0.000000000000000000 ) ) ;
#10688=EDGE_CURVE ( 'NONE', #4963, #655, #2460, .T. ) ;
#10700=EDGE_CURVE ( 'NONE', #9191, #2419, #6057, .T. ) ;
#10713=DIRECTION ( 'NONE',  ( 0.000000000000000000, -1.000000000000000000, 1.370729058197317775E-18 ) ) ;
#10724=CARTESIAN_POINT ( 'NONE',  ( 46.89999999999997016, 90.00000000000000000, -10.00000000000000000 ) ) ;
#10730=DIRECTION ( 'NONE',  ( 0.000000000000000000, 0.000000000000000000, -1.000000000000000000 ) ) ;
#10733=CARTESIAN_POINT ( 'NONE',  ( 38.50000000000000711, 90.00000000000000000, 6.000000000000000000 ) ) ;
#10734=ORIENTED_EDGE ( 'NONE', *, *, #705, .T. ) ;
#10741=EDGE_CURVE ( 'NONE', #294, #408, #4817, .T. ) ;
#10745=VECTOR ( 'NONE', #5854, 1000.000000000000000 ) ;
#10746=EDGE_CURVE ( 'NONE', #9892, #7985, #12270, .T. ) ;
#10762=CARTESIAN_POINT ( 'NONE',  ( 34.25000000000000000, 93.26496554346289258, 4.800000000000000711 ) ) ;
#10767=AXIS2_PLACEMENT_3D ( 'NONE', #6998, #1236, #10263 ) ;
#10782=ORIENTED_EDGE ( 'NONE', *, *, #3925, .F. ) ;
#10784=DIRECTION ( 'NONE',  ( -0.000000000000000000, -0.000000000000000000, 1.000000000000000000 ) ) ;
#10790=DIRECTION ( 'NONE',  ( 0.000000000000000000, 0.000000000000000000, -1.000000000000000000 ) ) ;
#10793=DIRECTION ( 'NONE',  ( -1.000000000000000000, 0.000000000000000000, 0.000000000000000000 ) ) ;
#10880=ORIENTED_EDGE ( 'NONE', *, *, #8124, .F. ) ;
#10886=CARTESIAN_POINT ( 'NONE',  ( 34.25000000000000000, 92.49999999999998579, -8.000000000000000000 ) ) ;
#10888=DIRECTION ( 'NONE',  ( -1.000000000000000000, 0.000000000000000000, 0.000000000000000000 ) ) ;
#10904=FACE_OUTER_BOUND ( 'NONE', #9101, .T. ) ;
#10915=ORIENTED_EDGE ( 'NONE', *, *, #7392, .T. ) ;
#10917=VERTEX_POINT ( 'NONE', #5781 ) ;
#10918=CYLINDRICAL_SURFACE ( 'NONE', #5843, 3.500000000000003109 ) ;
#10919=ORIENTED_EDGE ( 'NONE', *, *, #5911, .F. ) ;
#10936=DIRECTION ( 'NONE',  ( -5.624500927088228034E-17, 1.370729058197317968E-18, 1.000000000000000000 ) ) ;
#10952=VECTOR ( 'NONE', #668, 1000.000000000000000 ) ;
#10956=CARTESIAN_POINT ( 'NONE',  ( 31.99902028769960438, 88.51116798584881451, -3.000000000000000000 ) ) ;
#10966=CARTESIAN_POINT ( 'NONE',  ( 52.49999999999996447, 94.00000000000000000, -10.00000000000000000 ) ) ;
#10970=FACE_OUTER_BOUND ( 'NONE', #2253, .T. ) ;
#10975=CARTESIAN_POINT ( 'NONE',  ( 34.25000000000000000, 93.41869858279433458, 6.000000000000000000 ) ) ;
#10989=DIRECTION ( 'NONE',  ( -0.3262398754384820410, 0.9452870165584015272, 0.000000000000000000 ) ) ;
#10996=CARTESIAN_POINT ( 'NONE',  ( 35.00000000000000000, 90.00000000000000000, 4.000000000000000000 ) ) ;
#11008=PLANE ( 'NONE',  #165 ) ;
#11010=CIRCLE ( 'NONE', #3515, 3.350000000000003642 ) ;
#11013=EDGE_CURVE ( 'NONE', #29, #7014, #4022, .T. ) ;
#11025=EDGE_CURVE ( 'NONE', #4194, #11844, #2055, .T. ) ;
#11026=CARTESIAN_POINT ( 'NONE',  ( 31.50000000000000000, 90.00000000000000000, 4.800000000000000711 ) ) ;
#11028=ADVANCED_FACE ( 'NONE', ( #11864 ), #4149, .T. ) ;
#11038=CARTESIAN_POINT ( 'NONE',  ( 35.00000000000000000, 90.00000000000000000, -3.000000000000000000 ) ) ;
#11048=CARTESIAN_POINT ( 'NONE',  ( 38.50000000000000711, 90.00000000000000000, 4.800000000000000711 ) ) ;
#11056=( NAMED_UNIT ( * ) SI_UNIT ( $, .STERADIAN. ) SOLID_ANGLE_UNIT ( ) );
#11062=DIRECTION ( 'NONE',  ( -0.000000000000000000, -0.000000000000000000, -1.000000000000000000 ) ) ;
#11064=ORIENTED_EDGE ( 'NONE', *, *, #8706, .T. ) ;
#11084=ORIENTED_EDGE ( 'NONE', *, *, #11956, .F. ) ;
#11094=LINE ( 'NONE', #12218, #4812 ) ;
#11098=ORIENTED_EDGE ( 'NONE', *, *, #10741, .T. ) ;
#11113=CARTESIAN_POINT ( 'NONE',  ( 48.49999999999995737, 86.00000000000000000, -8.000000000000000000 ) ) ;
#11119=CARTESIAN_POINT ( 'NONE',  ( 35.75000000000000711, 93.41869858279433458, -8.000000000000000000 ) ) ;
#11127=VERTEX_POINT ( 'NONE', #11205 ) ;
#11128=DIRECTION ( 'NONE',  ( 0.000000000000000000, -0.000000000000000000, 1.000000000000000000 ) ) ;
#11149=DIRECTION ( 'NONE',  ( -1.000000000000000000, 0.000000000000000000, 0.000000000000000000 ) ) ;
#11151=VECTOR ( 'NONE', #5518, 1000.000000000000000 ) ;
#11172=CARTESIAN_POINT ( 'NONE',  ( 32.09707732552327286, 88.32801317409231956, -3.800000000000000266 ) ) ;
#11174=ORIENTED_EDGE ( 'NONE', *, *, #8951, .F. ) ;
#11176=EDGE_LOOP ( 'NONE', ( #8042, #1469, #12231, #9599, #11856, #1231 ) ) ;
#11183=VECTOR ( 'NONE', #11407, 1000.000000000000000 ) ;
#11188=CIRCLE ( 'NONE', #4510, 10.00000000000000178 ) ;
#11193=( NAMED_UNIT ( * ) SI_UNIT ( $, .STERADIAN. ) SOLID_ANGLE_UNIT ( ) );
#11195=FACE_OUTER_BOUND ( 'NONE', #1746, .T. ) ;
#11196=ORIENTED_EDGE ( 'NONE', *, *, #6536, .F. ) ;
#11200=CARTESIAN_POINT ( 'NONE',  ( 35.75000000000000711, 93.26496554346289258, -3.799999999999999822 ) ) ;
#11205=CARTESIAN_POINT ( 'NONE',  ( 31.65768047819777919, 88.96129878493390208, 4.000000000000000000 ) ) ;
#11209=DIRECTION ( 'NONE',  ( 0.000000000000000000, 0.000000000000000000, -1.000000000000000000 ) ) ;
#11212=CARTESIAN_POINT ( 'NONE',  ( 35.75000000000000711, 93.26496554346289258, -3.799999999999999822 ) ) ;
#11231=ORIENTED_EDGE ( 'NONE', *, *, #3443, .F. ) ;
#11241=VECTOR ( 'NONE', #1641, 1000.000000000000000 ) ;
#11257=VERTEX_POINT ( 'NONE', #3305 ) ;
#11268=DIRECTION ( 'NONE',  ( 0.000000000000000000, 0.000000000000000000, 1.000000000000000000 ) ) ;
#11284=VECTOR ( 'NONE', #3053, 1000.000000000000000 ) ;
#11290=LINE ( 'NONE', #8223, #8850 ) ;
#11297=ORIENTED_EDGE ( 'NONE', *, *, #4120, .T. ) ;
#11299=DIRECTION ( 'NONE',  ( 1.000000000000000000, 0.000000000000000000, 0.000000000000000000 ) ) ;
#11317=SURFACE_SIDE_STYLE ('',( #3226 ) ) ;
#11330=LINE ( 'NONE', #2448, #9540 ) ;
#11334=CARTESIAN_POINT ( 'NONE',  ( 35.00000000000000000, 90.00000000000000000, 6.000000000000000000 ) ) ;
#11343=DIRECTION ( 'NONE',  ( -5.624500927088228034E-17, 1.370729058197317775E-18, 1.000000000000000000 ) ) ;
#11358=CARTESIAN_POINT ( 'NONE',  ( 21.49999999999998579, 90.00000000000000000, -10.00000000000000000 ) ) ;
#11362=DIRECTION ( 'NONE',  ( 1.000000000000000000, 0.000000000000000000, 0.000000000000000000 ) ) ;
#11376=EDGE_CURVE ( 'NONE', #11634, #237, #2546, .T. ) ;
#11381=ORIENTED_EDGE ( 'NONE', *, *, #12451, .F. ) ;
#11383=VECTOR ( 'NONE', #971, 1000.000000000000000 ) ;
#11407=DIRECTION ( 'NONE',  ( 0.000000000000000000, 0.000000000000000000, -1.000000000000000000 ) ) ;
#11416=AXIS2_PLACEMENT_3D ( 'NONE', #5521, #7490, #12334 ) ;
#11459=ORIENTED_EDGE ( 'NONE', *, *, #1964, .T. ) ;
#11483=EDGE_CURVE ( 'NONE', #5120, #7980, #6083, .T. ) ;
#11502=CARTESIAN_POINT ( 'NONE',  ( 46.89999999999997016, 90.00000000000000000, -10.00000000000000178 ) ) ;
#11504=DIRECTION ( 'NONE',  ( -1.000000000000000000, 0.000000000000000000, 0.000000000000000000 ) ) ;
#11507=ORIENTED_EDGE ( 'NONE', *, *, #3660, .F. ) ;
#11514=VERTEX_POINT ( 'NONE', #1043 ) ;
#11516=DIRECTION ( 'NONE',  ( 0.000000000000000000, 1.000000000000000000, 0.000000000000000000 ) ) ;
#11536=CARTESIAN_POINT ( 'NONE',  ( 35.75000000000000711, 92.49999999999998579, 4.800000000000000711 ) ) ;
#11545=ORIENTED_EDGE ( 'NONE', *, *, #5579, .F. ) ;
#11553=DIRECTION ( 'NONE',  ( 0.000000000000000000, -0.000000000000000000, 1.000000000000000000 ) ) ;
#11557=DIRECTION ( 'NONE',  ( -1.000000000000000000, 0.000000000000000000, 0.000000000000000000 ) ) ;
#11606=CARTESIAN_POINT ( 'NONE',  ( 35.75000000000000711, 92.49999999999998579, -9.802775637731997449 ) ) ;
#11612=AXIS2_PLACEMENT_3D ( 'NONE', #12778, #4798, #10377 ) ;
#11616=CARTESIAN_POINT ( 'NONE',  ( 35.75000000000000711, 92.49999999999998579, -3.799999999999999378 ) ) ;
#11624=LINE ( 'NONE', #12675, #115 ) ;
#11629=CARTESIAN_POINT ( 'NONE',  ( 21.49999999999998579, 90.00000000000000000, -8.000000000000000000 ) ) ;
#11630=CARTESIAN_POINT ( 'NONE',  ( 34.25000000000000000, 92.49999999999998579, 6.000000000000000000 ) ) ;
#11634=VERTEX_POINT ( 'NONE', #5361 ) ;
#11638=EDGE_CURVE ( 'NONE', #8631, #3957, #7267, .T. ) ;
#11647=VECTOR ( 'NONE', #9709, 1000.000000000000114 ) ;
#11649=EDGE_LOOP ( 'NONE', ( #3805, #10321, #9774, #5683 ) ) ;
#11656=AXIS2_PLACEMENT_3D ( 'NONE', #5429, #447, #583 ) ;
#11678=VECTOR ( 'NONE', #5962, 1000.000000000000000 ) ;
#11696=AXIS2_PLACEMENT_3D ( 'NONE', #3923, #5872, #8760 ) ;
#11701=LINE ( 'NONE', #769, #6896 ) ;
#11704=ORIENTED_EDGE ( 'NONE', *, *, #3180, .T. ) ;
#11710=FACE_OUTER_BOUND ( 'NONE', #2847, .T. ) ;
#11734=ORIENTED_EDGE ( 'NONE', *, *, #11956, .T. ) ;
#11738=EDGE_LOOP ( 'NONE', ( #10595, #9818 ) ) ;
#11739=FILL_AREA_STYLE ('',( #12729 ) ) ;
#11745=MANIFOLD_SOLID_BREP ( 'M3 Clearance Hole1', #699 ) ;
#11755=CARTESIAN_POINT ( 'NONE',  ( 31.99902028769960438, 88.51116798584881451, -3.800000000000000266 ) ) ;
#11758=CARTESIAN_POINT ( 'NONE',  ( 35.00000000000000000, 90.00000000000000000, -10.00000000000000000 ) ) ;
#11773=CARTESIAN_POINT ( 'NONE',  ( 34.25000000000000000, 92.49999999999998579, -9.802775637731997449 ) ) ;
#11779=CARTESIAN_POINT ( 'NONE',  ( 31.86464806177570352, 88.44450386581220869, -3.799999999999999378 ) ) ;
#11783=EDGE_CURVE ( 'NONE', #3363, #5372, #1570, .T. ) ;
#11784=ORIENTED_EDGE ( 'NONE', *, *, #3180, .F. ) ;
#11799=CIRCLE ( 'NONE', #6366, 10.00000000000000178 ) ;
#11800=CARTESIAN_POINT ( 'NONE',  ( 35.00000000000000000, 90.00000000000000000, -3.000000000000000888 ) ) ;
#11801=ADVANCED_FACE ( 'NONE', ( #10970 ), #2883, .T. ) ;
#11819=ORIENTED_EDGE ( 'NONE', *, *, #10093, .F. ) ;
#11822=CARTESIAN_POINT ( 'NONE',  ( 35.00000000000000000, 90.00000000000000000, -3.799999999999999378 ) ) ;
#11830=PLANE ( 'NONE',  #12443 ) ;
#11834=CIRCLE ( 'NONE', #6186, 3.500000000000003109 ) ;
#11842=VECTOR ( 'NONE', #7762, 1000.000000000000114 ) ;
#11844=VERTEX_POINT ( 'NONE', #1956 ) ;
#11851=CIRCLE ( 'NONE', #7251, 3.349999999999995204 ) ;
#11856=ORIENTED_EDGE ( 'NONE', *, *, #3497, .T. ) ;
#11864=FACE_OUTER_BOUND ( 'NONE', #9034, .T. ) ;
#11870=CIRCLE ( 'NONE', #3941, 3.500000000000003109 ) ;
#11878=DIRECTION ( 'NONE',  ( -0.000000000000000000, -0.000000000000000000, -1.000000000000000000 ) ) ;
#11880=VERTEX_POINT ( 'NONE', #6924 ) ;
#11887=CARTESIAN_POINT ( 'NONE',  ( 32.09707732552327286, 88.32801317409231956, -3.800000000000000266 ) ) ;
#11900=DIRECTION ( 'NONE',  ( -5.624500927088228034E-17, 1.370729058197317775E-18, 1.000000000000000000 ) ) ;
#11911=ORIENTED_EDGE ( 'NONE', *, *, #841, .T. ) ;
#11924=ORIENTED_EDGE ( 'NONE', *, *, #7084, .T. ) ;
#11927=ORIENTED_EDGE ( 'NONE', *, *, #8286, .T. ) ;
#11937=PLANE ( 'NONE',  #8163 ) ;
#11939=ADVANCED_FACE ( 'NONE', ( #10498 ), #7556, .T. ) ;
#11942=VERTEX_POINT ( 'NONE', #409 ) ;
#11943=CARTESIAN_POINT ( 'NONE',  ( 34.25000000000000000, 93.41869858279433458, 6.000000000000000000 ) ) ;
#11956=EDGE_CURVE ( 'NONE', #12821, #3363, #6503, .T. ) ;
#12004=CARTESIAN_POINT ( 'NONE',  ( 48.49999999999995737, 90.00000000000000000, -10.00000000000000000 ) ) ;
#12019=EDGE_LOOP ( 'NONE', ( #7020, #9556, #578, #5698 ) ) ;
#12024=ORIENTED_EDGE ( 'NONE', *, *, #8706, .F. ) ;
#12027=ORIENTED_EDGE ( 'NONE', *, *, #5911, .T. ) ;
#12034=ORIENTED_EDGE ( 'NONE', *, *, #10700, .F. ) ;
#12036=ORIENTED_EDGE ( 'NONE', *, *, #10071, .F. ) ;
#12041=EDGE_LOOP ( 'NONE', ( #299, #8993, #11459, #1797 ) ) ;
#12050=ORIENTED_EDGE ( 'NONE', *, *, #12730, .F. ) ;
#12052=LINE ( 'NONE', #3099, #1877 ) ;
#12061=ORIENTED_EDGE ( 'NONE', *, *, #2653, .F. ) ;
#12066=VECTOR ( 'NONE', #6298, 1000.000000000000000 ) ;
#12072=CARTESIAN_POINT ( 'NONE',  ( 35.00000000000000000, 90.00000000000000000, 6.000000000000000000 ) ) ;
#12074=ORIENTED_EDGE ( 'NONE', *, *, #8856, .F. ) ;
#12083=VERTEX_POINT ( 'NONE', #9571 ) ;
#12084=DIRECTION ( 'NONE',  ( -1.000000000000000000, 0.000000000000000000, 0.000000000000000000 ) ) ;
#12096=VECTOR ( 'NONE', #7420, 1000.000000000000000 ) ;
#12115=CARTESIAN_POINT ( 'NONE',  ( 35.00000000000000000, 90.00000000000000000, -3.799999999999999822 ) ) ;
#12126=DIRECTION ( 'NONE',  ( -0.000000000000000000, -0.000000000000000000, -1.000000000000000000 ) ) ;
#12135=CARTESIAN_POINT ( 'NONE',  ( 44.16515138991168499, 86.00000000000000000, -18.00000000000000355 ) ) ;
#12137=ADVANCED_FACE ( 'NONE', ( #660 ), #4791, .T. ) ;
#12145=VECTOR ( 'NONE', #7989, 1000.000000000000000 ) ;
#12152=VERTEX_POINT ( 'NONE', #7795 ) ;
#12159=ORIENTED_EDGE ( 'NONE', *, *, #310, .T. ) ;
#12175=CARTESIAN_POINT ( 'NONE',  ( 35.75000000000000711, 92.49999999999998579, 6.000000000000000000 ) ) ;
#12179=CARTESIAN_POINT ( 'NONE',  ( 0.000000000000000000, 0.000000000000000000, -10.00000000000000000 ) ) ;
#12188=AXIS2_PLACEMENT_3D ( 'NONE', #5115, #10222, #2185 ) ;
#12195=EDGE_CURVE ( 'NONE', #655, #216, #21, .T. ) ;
#12200=DIRECTION ( 'NONE',  ( 0.000000000000000000, 0.000000000000000000, -1.000000000000000000 ) ) ;
#12207=VERTEX_POINT ( 'NONE', #2900 ) ;
#12218=CARTESIAN_POINT ( 'NONE',  ( 31.96709571323326671, 88.25314809233525182, 6.000000000000000000 ) ) ;
#12227=AXIS2_PLACEMENT_3D ( 'NONE', #2145, #5400, #6319 ) ;
#12230=VECTOR ( 'NONE', #5289, 1000.000000000000000 ) ;
#12231=ORIENTED_EDGE ( 'NONE', *, *, #7619, .T. ) ;
#12233=ORIENTED_EDGE ( 'NONE', *, *, #12239, .T. ) ;
#12239=EDGE_CURVE ( 'NONE', #4447, #7980, #8201, .T. ) ;
#12241=EDGE_CURVE ( 'NONE', #9627, #4130, #7928, .T. ) ;
#12259=VECTOR ( 'NONE', #12126, 1000.000000000000000 ) ;
#12270=LINE ( 'NONE', #7296, #1042 ) ;
#12272=ORIENTED_EDGE ( 'NONE', *, *, #9024, .T. ) ;
#12273=DIRECTION ( 'NONE',  ( -0.000000000000000000, -0.000000000000000000, -1.000000000000000000 ) ) ;
#12282=DIRECTION ( 'NONE',  ( -0.000000000000000000, -0.000000000000000000, -1.000000000000000000 ) ) ;
#12297=VERTEX_POINT ( 'NONE', #5240 ) ;
#12313=ORIENTED_EDGE ( 'NONE', *, *, #931, .T. ) ;
#12322=DIRECTION ( 'NONE',  ( -0.000000000000000000, -1.000000000000000000, -0.000000000000000000 ) ) ;
#12334=DIRECTION ( 'NONE',  ( 1.000000000000000000, 0.000000000000000000, -0.000000000000000000 ) ) ;
#12343=CARTESIAN_POINT ( 'NONE',  ( 35.75000000000000711, 93.41869858279433458, -3.799999999999999378 ) ) ;
#12349=ORIENTED_EDGE ( 'NONE', *, *, #8879, .F. ) ;
#12352=ORIENTED_EDGE ( 'NONE', *, *, #10102, .T. ) ;
#12366=FACE_OUTER_BOUND ( 'NONE', #1158, .T. ) ;
#12378=ORIENTED_EDGE ( 'NONE', *, *, #867, .T. ) ;
#12379=VECTOR ( 'NONE', #9936, 1000.000000000000227 ) ;
#12395=ADVANCED_FACE ( 'NONE', ( #4455 ), #5171, .F. ) ;
#12396=EDGE_CURVE ( 'NONE', #7515, #2123, #8188, .T. ) ;
#12402=DIRECTION ( 'NONE',  ( 0.000000000000000000, -0.000000000000000000, 1.000000000000000000 ) ) ;
#12408=ORIENTED_EDGE ( 'NONE', *, *, #12730, .T. ) ;
#12412=VERTEX_POINT ( 'NONE', #6476 ) ;
#12414=CARTESIAN_POINT ( 'NONE',  ( 35.00000000000000000, 90.00000000000000000, 4.000000000000000000 ) ) ;
#12421=PRODUCT_DEFINITION_SHAPE ( 'NONE', 'NONE',  #2349 ) ;
#12423=AXIS2_PLACEMENT_3D ( 'NONE', #9638, #535, #7419 ) ;
#12425=DIRECTION ( 'NONE',  ( -0.3262398754384822630, 0.9452870165584014162, 0.000000000000000000 ) ) ;
#12439=DIRECTION ( 'NONE',  ( 0.000000000000000000, 0.000000000000000000, -1.000000000000000000 ) ) ;
#12443=AXIS2_PLACEMENT_3D ( 'NONE', #10966, #9070, #8942 ) ;
#12451=EDGE_CURVE ( 'NONE', #12152, #4194, #2779, .T. ) ;
#12456=VECTOR ( 'NONE', #3582, 1000.000000000000114 ) ;
#12461=PLANE ( 'NONE',  #10575 ) ;
#12467=DIRECTION ( 'NONE',  ( 1.000000000000000000, 0.000000000000000000, 0.000000000000000000 ) ) ;
#12479=ORIENTED_EDGE ( 'NONE', *, *, #7923, .F. ) ;
#12485=ORIENTED_EDGE ( 'NONE', *, *, #3228, .F. ) ;
#12486=EDGE_CURVE ( 'NONE', #2419, #11257, #4904, .T. ) ;
#12489=ORIENTED_EDGE ( 'NONE', *, *, #6577, .F. ) ;
#12497=DIRECTION ( 'NONE',  ( -0.000000000000000000, -0.000000000000000000, -1.000000000000000000 ) ) ;
#12505=DIRECTION ( 'NONE',  ( 0.4719909656437444867, -0.8816033849473842166, 0.000000000000000000 ) ) ;
#12506=FACE_BOUND ( 'NONE', #8894, .T. ) ;
#12511=VECTOR ( 'NONE', #7122, 1000.000000000000000 ) ;
#12535=CARTESIAN_POINT ( 'NONE',  ( 35.00000000000000000, 90.00000000000000000, -18.00000000000000355 ) ) ;
#12542=ADVANCED_FACE ( 'NONE', ( #2885 ), #4841, .T. ) ;
#12543=CARTESIAN_POINT ( 'NONE',  ( 38.50000000000000711, 90.00000000000000000, 6.000000000000000000 ) ) ;
#12548=CIRCLE ( 'NONE', #1257, 3.500000000000003109 ) ;
#12554=ORIENTED_EDGE ( 'NONE', *, *, #12920, .T. ) ;
#12555=EDGE_CURVE ( 'NONE', #12562, #9627, #9030, .T. ) ;
#12557=DIRECTION ( 'NONE',  ( 0.4719909656437442647, -0.8816033849473842166, 2.775557561595757269E-17 ) ) ;
#12562=VERTEX_POINT ( 'NONE', #10059 ) ;
#12574=LINE ( 'NONE', #5493, #2273 ) ;
#12589=EDGE_CURVE ( 'NONE', #12297, #11127, #6798, .T. ) ;
#12601=CIRCLE ( 'NONE', #2148, 3.500000000000003109 ) ;
#12608=VERTEX_POINT ( 'NONE', #7977 ) ;
#12612=ORIENTED_EDGE ( 'NONE', *, *, #8720, .F. ) ;
#12618=DIRECTION ( 'NONE',  ( -5.624500927088228034E-17, 1.370729058197317775E-18, 1.000000000000000000 ) ) ;
#12633=EDGE_CURVE ( 'NONE', #2177, #11634, #4036, .T. ) ;
#12635=DIRECTION ( 'NONE',  ( 0.000000000000000000, 0.000000000000000000, 1.000000000000000000 ) ) ;
#12636=CIRCLE ( 'NONE', #4695, 3.349999999999995204 ) ;
#12639=ORIENTED_EDGE ( 'NONE', *, *, #1888, .F. ) ;
#12650=CARTESIAN_POINT ( 'NONE',  ( 34.25000000000000000, 93.26496554346289258, 4.000000000000000000 ) ) ;
#12669=DIRECTION ( 'NONE',  ( 0.000000000000000000, -1.000000000000000000, 0.000000000000000000 ) ) ;
#12675=CARTESIAN_POINT ( 'NONE',  ( 48.49999999999995737, 86.00000000000000000, -10.00000000000000000 ) ) ;
#12689=CARTESIAN_POINT ( 'NONE',  ( 21.49999999999998579, 94.00000000000000000, -8.000000000000000000 ) ) ;
#12699=CIRCLE ( 'NONE', #4136, 3.500000000000003109 ) ;
#12702=ORIENTED_EDGE ( 'NONE', *, *, #10688, .F. ) ;
#12705=EDGE_LOOP ( 'NONE', ( #8428, #3742, #3231, #6777 ) ) ;
#12715=VECTOR ( 'NONE', #285, 1000.000000000000000 ) ;
#12727=DIRECTION ( 'NONE',  ( -0.000000000000000000, -0.000000000000000000, 1.000000000000000000 ) ) ;
#12728=ORIENTED_EDGE ( 'NONE', *, *, #4873, .T. ) ;
#12729=FILL_AREA_STYLE_COLOUR ( '', #2589 ) ;
#12730=EDGE_CURVE ( 'NONE', #4783, #11942, #166, .T. ) ;
#12749=DIRECTION ( 'NONE',  ( -0.000000000000000000, -0.000000000000000000, -1.000000000000000000 ) ) ;
#12760=CIRCLE ( 'NONE', #7508, 3.500000000000003109 ) ;
#12773=DIRECTION ( 'NONE',  ( -0.3262398754384822630, 0.9452870165584014162, 0.000000000000000000 ) ) ;
#12775=EDGE_CURVE ( 'NONE', #10536, #8908, #1087, .T. ) ;
#12778=CARTESIAN_POINT ( 'NONE',  ( 35.00000000000000000, 90.00000000000000000, 6.000000000000000000 ) ) ;
#12782=DIRECTION ( 'NONE',  ( -5.624500927088228034E-17, 1.370729058197317775E-18, 1.000000000000000000 ) ) ;
#12805=DIRECTION ( 'NONE',  ( 1.000000000000000000, 0.000000000000000000, 0.000000000000000000 ) ) ;
#12807=ORIENTED_EDGE ( 'NONE', *, *, #10102, .F. ) ;
#12813=ORIENTED_EDGE ( 'NONE', *, *, #11638, .T. ) ;
#12821=VERTEX_POINT ( 'NONE', #5735 ) ;
#12835=DIRECTION ( 'NONE',  ( -1.000000000000000000, 0.000000000000000000, 0.000000000000000000 ) ) ;
#12844=CIRCLE ( 'NONE', #7417, 3.500000000000003109 ) ;
#12847=EDGE_LOOP ( 'NONE', ( #4600, #557, #1335, #1981 ) ) ;
#12849=DIRECTION ( 'NONE',  ( 1.000000000000000000, 0.000000000000000000, 0.000000000000000000 ) ) ;
#12855=AXIS2_PLACEMENT_3D ( 'NONE', #9396, #2409, #10250 ) ;
#12856=AXIS2_PLACEMENT_3D ( 'NONE', #6592, #2487, #10460 ) ;
#12863=CARTESIAN_POINT ( 'NONE',  ( 35.75000000000000711, 93.41869858279433458, 6.000000000000000000 ) ) ;
#12868=CIRCLE ( 'NONE', #4311, 3.500000000000003109 ) ;
#12876=LINE ( 'NONE', #9735, #4792 ) ;
#12888=DIRECTION ( 'NONE',  ( -5.624500927088228034E-17, 1.370729058197317775E-18, 1.000000000000000000 ) ) ;
#12889=CYLINDRICAL_SURFACE ( 'NONE', #9988, 3.350000000000003642 ) ;
#12900=VECTOR ( 'NONE', #6634, 1000.000000000000000 ) ;
#12906=EDGE_CURVE ( 'NONE', #6452, #9676, #12601, .T. ) ;
#12920=EDGE_CURVE ( 'NONE', #9660, #11844, #8026, .T. ) ;
#12929=LINE ( 'NONE', #10956, #11842 ) ;
#12940=CARTESIAN_POINT ( 'NONE',  ( 35.00000000000000000, 90.00000000000000000, 4.800000000000000711 ) ) ;
#12949=CARTESIAN_POINT ( 'NONE',  ( 35.00000000000000000, 90.00000000000000000, -3.799999999999999822 ) ) ;
#12954=ORIENTED_EDGE ( 'NONE', *, *, #5063, .T. ) ;
#13010=COLOUR_RGB('Off White',0.89,0.88,0.83);
#13011=FILL_AREA_STYLE_COLOUR('',#13010);
#13012=FILL_AREA_STYLE('',(#13011));
#13013=SURFACE_STYLE_FILL_AREA(#13012);
#13014=SURFACE_SIDE_STYLE('',(#13013));
#13015=SURFACE_STYLE_USAGE(.BOTH.,#13014);
#13016=PRESENTATION_STYLE_ASSIGNMENT((#13015));
ENDSEC;
END-ISO-10303-21;
